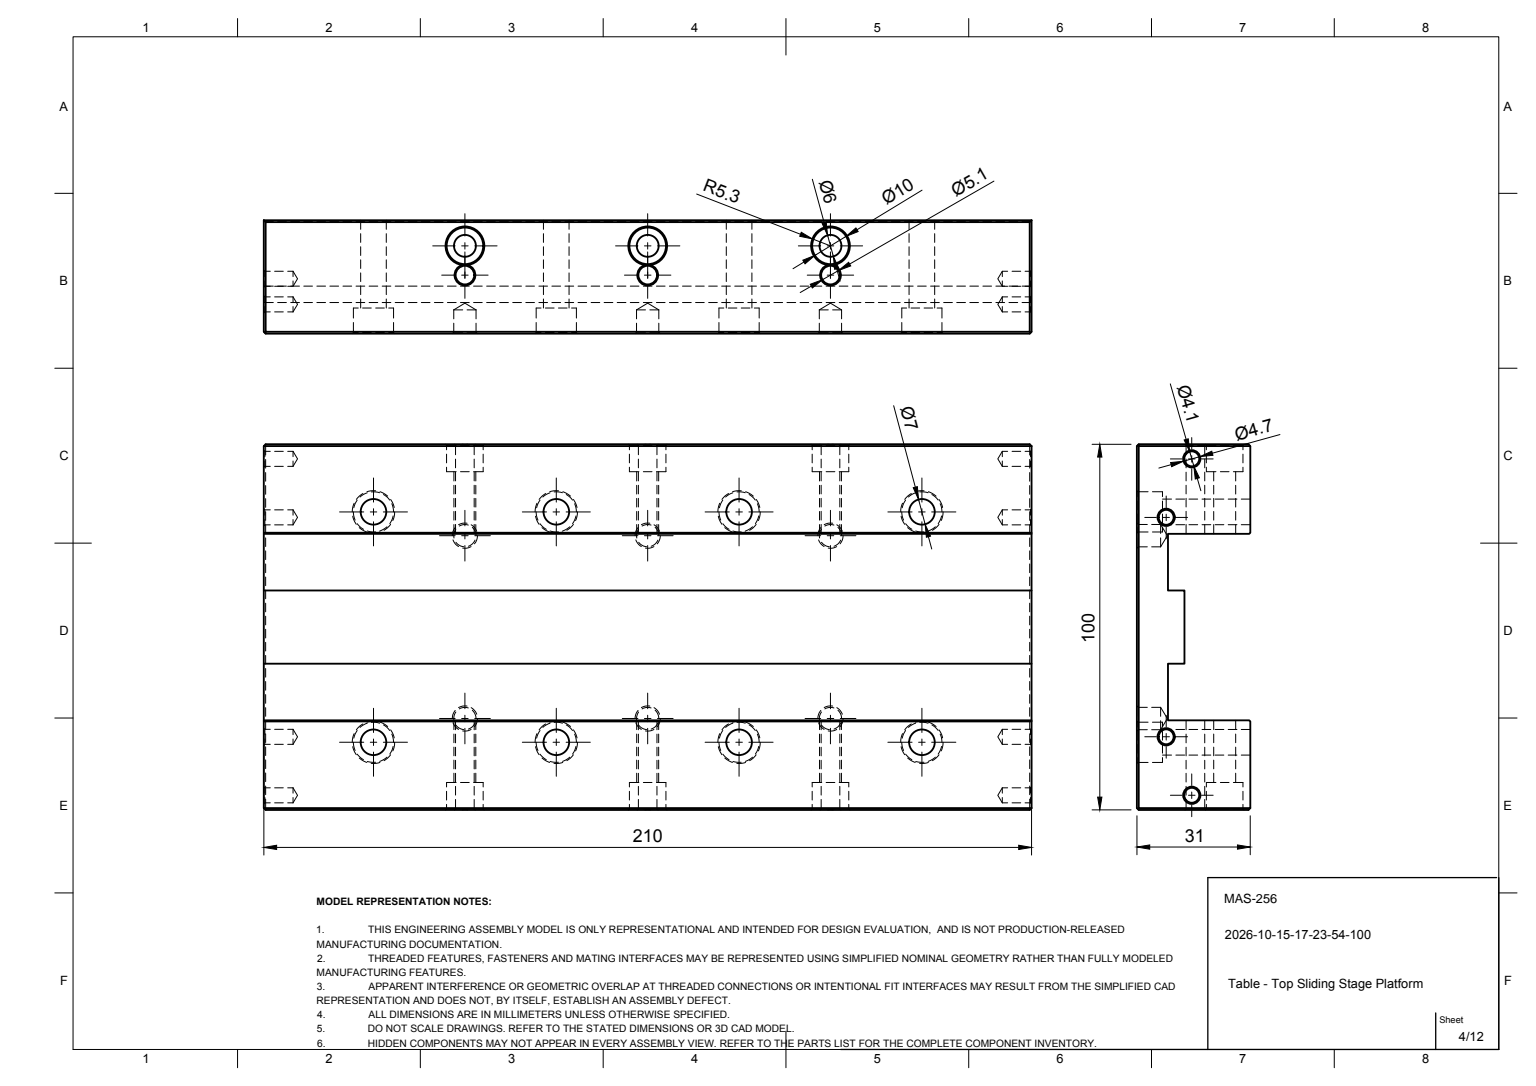
ISO-10303-21;
HEADER;
/* Generated by software containing ST-Developer
 * from STEP Tools, Inc. (www.steptools.com) 
 */

FILE_DESCRIPTION(
/* description */ (''),
/* implementation_level */ '2;1');

FILE_NAME(
/* name */ 'Table - Top Sliding Stage Platform.step',
/* time_stamp */ '2026-10-14T18:40:07-07:00',
/* author */ (''),
/* organization */ (''),
/* preprocessor_version */ 'ST-DEVELOPER v20.2',
/* originating_system */ 'Autodesk Translation Framework v15.15.0.0',
/* authorisation */ '');

FILE_SCHEMA (('AUTOMOTIVE_DESIGN { 1 0 10303 214 3 1 1 }'));
ENDSEC;

DATA;
#10=MECHANICAL_DESIGN_GEOMETRIC_PRESENTATION_REPRESENTATION('',(#832),#81040);
#402=B_SPLINE_CURVE_WITH_KNOTS('',3,(#20931,#20932,#20933,#20934,#20935,
#20936),.UNSPECIFIED.,.F.,.F.,(4,2,4),(1.66095691430957,1.73342009736541,
1.80588328042126),.UNSPECIFIED.);
#403=B_SPLINE_CURVE_WITH_KNOTS('',3,(#20957,#20958,#20959,#20960,#20961,
#20962),.UNSPECIFIED.,.F.,.F.,(4,2,4),(1.66095691430954,1.73342009736538,
1.80588328042123),.UNSPECIFIED.);
#404=B_SPLINE_CURVE_WITH_KNOTS('',3,(#20983,#20984,#20985,#20986,#20987,
#20988),.UNSPECIFIED.,.F.,.F.,(4,2,4),(1.66095691430954,1.73342009736541,
1.80588328042128),.UNSPECIFIED.);
#405=B_SPLINE_CURVE_WITH_KNOTS('',3,(#21051,#21052,#21053,#21054,#21055,
#21056),.UNSPECIFIED.,.F.,.F.,(4,2,4),(1.66095691430955,1.73342009736539,
1.80588328042123),.UNSPECIFIED.);
#406=B_SPLINE_CURVE_WITH_KNOTS('',3,(#21077,#21078,#21079,#21080,#21081,
#21082),.UNSPECIFIED.,.F.,.F.,(4,2,4),(1.66095691430953,1.73342009736537,
1.80588328042121),.UNSPECIFIED.);
#407=B_SPLINE_CURVE_WITH_KNOTS('',3,(#21103,#21104,#21105,#21106,#21107,
#21108),.UNSPECIFIED.,.F.,.F.,(4,2,4),(1.66095691430952,1.73342009736539,
1.80588328042126),.UNSPECIFIED.);
#812=SHAPE_REPRESENTATION_RELATIONSHIP('SRR','None',#81131,#822);
#822=ADVANCED_BREP_SHAPE_REPRESENTATION('',(#842),#81031);
#832=STYLED_ITEM('',(#81190),#842);
#842=MANIFOLD_SOLID_BREP('Body1',#15085);
#867=CYLINDRICAL_SURFACE('',#15336,2.55000000000001);
#868=CYLINDRICAL_SURFACE('',#15346,2.55000000000001);
#869=CYLINDRICAL_SURFACE('',#15356,2.55);
#870=CYLINDRICAL_SURFACE('',#15359,5.);
#871=CYLINDRICAL_SURFACE('',#15361,5.);
#872=CYLINDRICAL_SURFACE('',#15363,5.);
#873=CYLINDRICAL_SURFACE('',#15371,3.);
#874=CYLINDRICAL_SURFACE('',#15373,3.00000000000001);
#875=CYLINDRICAL_SURFACE('',#15375,3.00000000000001);
#876=CYLINDRICAL_SURFACE('',#15385,2.55000000000001);
#877=CYLINDRICAL_SURFACE('',#15395,2.55000000000001);
#878=CYLINDRICAL_SURFACE('',#15405,2.55);
#879=CYLINDRICAL_SURFACE('',#15408,5.);
#880=CYLINDRICAL_SURFACE('',#15410,5.);
#881=CYLINDRICAL_SURFACE('',#15412,5.);
#882=CYLINDRICAL_SURFACE('',#15420,3.);
#883=CYLINDRICAL_SURFACE('',#15422,3.00000000000001);
#884=CYLINDRICAL_SURFACE('',#15424,3.00000000000001);
#885=CYLINDRICAL_SURFACE('',#15433,2.05);
#886=CYLINDRICAL_SURFACE('',#15438,2.05);
#887=CYLINDRICAL_SURFACE('',#15443,2.05);
#888=CYLINDRICAL_SURFACE('',#15448,2.05);
#889=CYLINDRICAL_SURFACE('',#15462,2.05);
#890=CYLINDRICAL_SURFACE('',#15467,2.05);
#891=CYLINDRICAL_SURFACE('',#15472,2.05);
#892=CYLINDRICAL_SURFACE('',#15477,2.05);
#893=CYLINDRICAL_SURFACE('',#15501,3.05);
#894=CYLINDRICAL_SURFACE('',#15505,3.05);
#895=CYLINDRICAL_SURFACE('',#15509,3.05);
#896=CYLINDRICAL_SURFACE('',#15513,3.05);
#897=CYLINDRICAL_SURFACE('',#15517,3.05);
#898=CYLINDRICAL_SURFACE('',#15521,3.05);
#899=CYLINDRICAL_SURFACE('',#15531,5.50000000000001);
#900=CYLINDRICAL_SURFACE('',#15535,5.50000000000001);
#901=CYLINDRICAL_SURFACE('',#15539,5.5);
#902=CYLINDRICAL_SURFACE('',#15543,5.50000000000001);
#903=CYLINDRICAL_SURFACE('',#15547,5.5);
#904=CYLINDRICAL_SURFACE('',#15551,5.50000000000001);
#905=CYLINDRICAL_SURFACE('',#15555,5.50000000000001);
#906=CYLINDRICAL_SURFACE('',#15559,5.50000000000001);
#907=CYLINDRICAL_SURFACE('',#15577,3.50000000000001);
#908=CYLINDRICAL_SURFACE('',#15579,3.5);
#909=CYLINDRICAL_SURFACE('',#15581,3.5);
#910=CYLINDRICAL_SURFACE('',#15583,3.5);
#911=CYLINDRICAL_SURFACE('',#15585,3.5);
#912=CYLINDRICAL_SURFACE('',#15587,3.5);
#913=CYLINDRICAL_SURFACE('',#15589,3.5);
#914=CYLINDRICAL_SURFACE('',#15591,3.50000000000001);
#1107=FACE_BOUND('',#2455,.T.);
#1108=FACE_BOUND('',#2456,.T.);
#1109=FACE_BOUND('',#2457,.T.);
#1110=FACE_BOUND('',#2462,.T.);
#1111=FACE_BOUND('',#2464,.T.);
#1112=FACE_BOUND('',#2466,.T.);
#1113=FACE_BOUND('',#2480,.T.);
#1114=FACE_BOUND('',#2481,.T.);
#1115=FACE_BOUND('',#2482,.T.);
#1116=FACE_BOUND('',#2487,.T.);
#1117=FACE_BOUND('',#2489,.T.);
#1118=FACE_BOUND('',#2491,.T.);
#1119=FACE_BOUND('',#2497,.T.);
#1120=FACE_BOUND('',#2498,.T.);
#1121=FACE_BOUND('',#2499,.T.);
#1122=FACE_BOUND('',#2500,.T.);
#1123=FACE_BOUND('',#2514,.T.);
#1124=FACE_BOUND('',#2515,.T.);
#1125=FACE_BOUND('',#2516,.T.);
#1126=FACE_BOUND('',#2517,.T.);
#1127=FACE_BOUND('',#2531,.T.);
#1128=FACE_BOUND('',#2532,.T.);
#1129=FACE_BOUND('',#2533,.T.);
#1130=FACE_BOUND('',#2534,.T.);
#1131=FACE_BOUND('',#2535,.T.);
#1132=FACE_BOUND('',#2536,.T.);
#1133=FACE_BOUND('',#2537,.T.);
#1134=FACE_BOUND('',#2538,.T.);
#1135=FACE_BOUND('',#2539,.T.);
#1136=FACE_BOUND('',#2540,.T.);
#1137=FACE_BOUND('',#2541,.T.);
#1138=FACE_BOUND('',#2542,.T.);
#1139=FACE_BOUND('',#2543,.T.);
#1140=FACE_BOUND('',#2544,.T.);
#1141=FACE_BOUND('',#2579,.T.);
#1142=FACE_BOUND('',#2581,.T.);
#1143=FACE_BOUND('',#2583,.T.);
#1144=FACE_BOUND('',#2585,.T.);
#1145=FACE_BOUND('',#2587,.T.);
#1146=FACE_BOUND('',#2589,.T.);
#1147=FACE_BOUND('',#2591,.T.);
#1148=FACE_BOUND('',#2593,.T.);
#1149=FACE_BOUND('',#2613,.T.);
#1150=FACE_BOUND('',#2614,.T.);
#1151=FACE_BOUND('',#2615,.T.);
#1152=FACE_BOUND('',#2616,.T.);
#1153=FACE_BOUND('',#2619,.T.);
#1154=FACE_BOUND('',#2620,.T.);
#1155=FACE_BOUND('',#2621,.T.);
#1156=FACE_BOUND('',#2622,.T.);
#1157=FACE_BOUND('',#2623,.T.);
#1158=FACE_BOUND('',#2624,.T.);
#1159=FACE_BOUND('',#2627,.T.);
#1160=FACE_BOUND('',#2628,.T.);
#1161=FACE_BOUND('',#2629,.T.);
#1162=FACE_BOUND('',#2630,.T.);
#1163=FACE_BOUND('',#2632,.T.);
#1164=FACE_BOUND('',#2633,.T.);
#1165=FACE_BOUND('',#2634,.T.);
#1166=FACE_BOUND('',#2635,.T.);
#1167=FACE_BOUND('',#2636,.T.);
#1168=FACE_BOUND('',#2637,.T.);
#1243=PLANE('',#15358);
#1244=PLANE('',#15365);
#1245=PLANE('',#15367);
#1246=PLANE('',#15369);
#1247=PLANE('',#15407);
#1248=PLANE('',#15414);
#1249=PLANE('',#15416);
#1250=PLANE('',#15418);
#1251=PLANE('',#15429);
#1252=PLANE('',#15458);
#1253=PLANE('',#15487);
#1254=PLANE('',#15561);
#1255=PLANE('',#15563);
#1256=PLANE('',#15565);
#1257=PLANE('',#15567);
#1258=PLANE('',#15569);
#1259=PLANE('',#15571);
#1260=PLANE('',#15573);
#1261=PLANE('',#15575);
#1262=PLANE('',#15593);
#1263=PLANE('',#15594);
#1264=PLANE('',#15595);
#1265=PLANE('',#15596);
#1266=PLANE('',#15597);
#1267=PLANE('',#15598);
#1268=PLANE('',#15599);
#1269=PLANE('',#15600);
#1270=PLANE('',#15601);
#1271=PLANE('',#15602);
#1272=PLANE('',#15603);
#1273=PLANE('',#15604);
#1274=PLANE('',#15605);
#1275=PLANE('',#15606);
#1276=PLANE('',#15607);
#1277=PLANE('',#15608);
#1278=PLANE('',#15609);
#1279=PLANE('',#15610);
#1280=PLANE('',#15611);
#1281=PLANE('',#15612);
#1282=PLANE('',#15613);
#1678=FACE_OUTER_BOUND('',#2445,.T.);
#1679=FACE_OUTER_BOUND('',#2446,.T.);
#1680=FACE_OUTER_BOUND('',#2447,.T.);
#1681=FACE_OUTER_BOUND('',#2448,.T.);
#1682=FACE_OUTER_BOUND('',#2449,.T.);
#1683=FACE_OUTER_BOUND('',#2450,.T.);
#1684=FACE_OUTER_BOUND('',#2451,.T.);
#1685=FACE_OUTER_BOUND('',#2452,.T.);
#1686=FACE_OUTER_BOUND('',#2453,.T.);
#1687=FACE_OUTER_BOUND('',#2454,.T.);
#1688=FACE_OUTER_BOUND('',#2458,.T.);
#1689=FACE_OUTER_BOUND('',#2459,.T.);
#1690=FACE_OUTER_BOUND('',#2460,.T.);
#1691=FACE_OUTER_BOUND('',#2461,.T.);
#1692=FACE_OUTER_BOUND('',#2463,.T.);
#1693=FACE_OUTER_BOUND('',#2465,.T.);
#1694=FACE_OUTER_BOUND('',#2467,.T.);
#1695=FACE_OUTER_BOUND('',#2468,.T.);
#1696=FACE_OUTER_BOUND('',#2469,.T.);
#1697=FACE_OUTER_BOUND('',#2470,.T.);
#1698=FACE_OUTER_BOUND('',#2471,.T.);
#1699=FACE_OUTER_BOUND('',#2472,.T.);
#1700=FACE_OUTER_BOUND('',#2473,.T.);
#1701=FACE_OUTER_BOUND('',#2474,.T.);
#1702=FACE_OUTER_BOUND('',#2475,.T.);
#1703=FACE_OUTER_BOUND('',#2476,.T.);
#1704=FACE_OUTER_BOUND('',#2477,.T.);
#1705=FACE_OUTER_BOUND('',#2478,.T.);
#1706=FACE_OUTER_BOUND('',#2479,.T.);
#1707=FACE_OUTER_BOUND('',#2483,.T.);
#1708=FACE_OUTER_BOUND('',#2484,.T.);
#1709=FACE_OUTER_BOUND('',#2485,.T.);
#1710=FACE_OUTER_BOUND('',#2486,.T.);
#1711=FACE_OUTER_BOUND('',#2488,.T.);
#1712=FACE_OUTER_BOUND('',#2490,.T.);
#1713=FACE_OUTER_BOUND('',#2492,.T.);
#1714=FACE_OUTER_BOUND('',#2493,.T.);
#1715=FACE_OUTER_BOUND('',#2494,.T.);
#1716=FACE_OUTER_BOUND('',#2495,.T.);
#1717=FACE_OUTER_BOUND('',#2496,.T.);
#1718=FACE_OUTER_BOUND('',#2501,.T.);
#1719=FACE_OUTER_BOUND('',#2502,.T.);
#1720=FACE_OUTER_BOUND('',#2503,.T.);
#1721=FACE_OUTER_BOUND('',#2504,.T.);
#1722=FACE_OUTER_BOUND('',#2505,.T.);
#1723=FACE_OUTER_BOUND('',#2506,.T.);
#1724=FACE_OUTER_BOUND('',#2507,.T.);
#1725=FACE_OUTER_BOUND('',#2508,.T.);
#1726=FACE_OUTER_BOUND('',#2509,.T.);
#1727=FACE_OUTER_BOUND('',#2510,.T.);
#1728=FACE_OUTER_BOUND('',#2511,.T.);
#1729=FACE_OUTER_BOUND('',#2512,.T.);
#1730=FACE_OUTER_BOUND('',#2513,.T.);
#1731=FACE_OUTER_BOUND('',#2518,.T.);
#1732=FACE_OUTER_BOUND('',#2519,.T.);
#1733=FACE_OUTER_BOUND('',#2520,.T.);
#1734=FACE_OUTER_BOUND('',#2521,.T.);
#1735=FACE_OUTER_BOUND('',#2522,.T.);
#1736=FACE_OUTER_BOUND('',#2523,.T.);
#1737=FACE_OUTER_BOUND('',#2524,.T.);
#1738=FACE_OUTER_BOUND('',#2525,.T.);
#1739=FACE_OUTER_BOUND('',#2526,.T.);
#1740=FACE_OUTER_BOUND('',#2527,.T.);
#1741=FACE_OUTER_BOUND('',#2528,.T.);
#1742=FACE_OUTER_BOUND('',#2529,.T.);
#1743=FACE_OUTER_BOUND('',#2530,.T.);
#1744=FACE_OUTER_BOUND('',#2545,.T.);
#1745=FACE_OUTER_BOUND('',#2546,.T.);
#1746=FACE_OUTER_BOUND('',#2547,.T.);
#1747=FACE_OUTER_BOUND('',#2548,.T.);
#1748=FACE_OUTER_BOUND('',#2549,.T.);
#1749=FACE_OUTER_BOUND('',#2550,.T.);
#1750=FACE_OUTER_BOUND('',#2551,.T.);
#1751=FACE_OUTER_BOUND('',#2552,.T.);
#1752=FACE_OUTER_BOUND('',#2553,.T.);
#1753=FACE_OUTER_BOUND('',#2554,.T.);
#1754=FACE_OUTER_BOUND('',#2555,.T.);
#1755=FACE_OUTER_BOUND('',#2556,.T.);
#1756=FACE_OUTER_BOUND('',#2557,.T.);
#1757=FACE_OUTER_BOUND('',#2558,.T.);
#1758=FACE_OUTER_BOUND('',#2559,.T.);
#1759=FACE_OUTER_BOUND('',#2560,.T.);
#1760=FACE_OUTER_BOUND('',#2561,.T.);
#1761=FACE_OUTER_BOUND('',#2562,.T.);
#1762=FACE_OUTER_BOUND('',#2563,.T.);
#1763=FACE_OUTER_BOUND('',#2564,.T.);
#1764=FACE_OUTER_BOUND('',#2565,.T.);
#1765=FACE_OUTER_BOUND('',#2566,.T.);
#1766=FACE_OUTER_BOUND('',#2567,.T.);
#1767=FACE_OUTER_BOUND('',#2568,.T.);
#1768=FACE_OUTER_BOUND('',#2569,.T.);
#1769=FACE_OUTER_BOUND('',#2570,.T.);
#1770=FACE_OUTER_BOUND('',#2571,.T.);
#1771=FACE_OUTER_BOUND('',#2572,.T.);
#1772=FACE_OUTER_BOUND('',#2573,.T.);
#1773=FACE_OUTER_BOUND('',#2574,.T.);
#1774=FACE_OUTER_BOUND('',#2575,.T.);
#1775=FACE_OUTER_BOUND('',#2576,.T.);
#1776=FACE_OUTER_BOUND('',#2577,.T.);
#1777=FACE_OUTER_BOUND('',#2578,.T.);
#1778=FACE_OUTER_BOUND('',#2580,.T.);
#1779=FACE_OUTER_BOUND('',#2582,.T.);
#1780=FACE_OUTER_BOUND('',#2584,.T.);
#1781=FACE_OUTER_BOUND('',#2586,.T.);
#1782=FACE_OUTER_BOUND('',#2588,.T.);
#1783=FACE_OUTER_BOUND('',#2590,.T.);
#1784=FACE_OUTER_BOUND('',#2592,.T.);
#1785=FACE_OUTER_BOUND('',#2594,.T.);
#1786=FACE_OUTER_BOUND('',#2595,.T.);
#1787=FACE_OUTER_BOUND('',#2596,.T.);
#1788=FACE_OUTER_BOUND('',#2597,.T.);
#1789=FACE_OUTER_BOUND('',#2598,.T.);
#1790=FACE_OUTER_BOUND('',#2599,.T.);
#1791=FACE_OUTER_BOUND('',#2600,.T.);
#1792=FACE_OUTER_BOUND('',#2601,.T.);
#1793=FACE_OUTER_BOUND('',#2602,.T.);
#1794=FACE_OUTER_BOUND('',#2603,.T.);
#1795=FACE_OUTER_BOUND('',#2604,.T.);
#1796=FACE_OUTER_BOUND('',#2605,.T.);
#1797=FACE_OUTER_BOUND('',#2606,.T.);
#1798=FACE_OUTER_BOUND('',#2607,.T.);
#1799=FACE_OUTER_BOUND('',#2608,.T.);
#1800=FACE_OUTER_BOUND('',#2609,.T.);
#1801=FACE_OUTER_BOUND('',#2610,.T.);
#1802=FACE_OUTER_BOUND('',#2611,.T.);
#1803=FACE_OUTER_BOUND('',#2612,.T.);
#1804=FACE_OUTER_BOUND('',#2617,.T.);
#1805=FACE_OUTER_BOUND('',#2618,.T.);
#1806=FACE_OUTER_BOUND('',#2625,.T.);
#1807=FACE_OUTER_BOUND('',#2626,.T.);
#1808=FACE_OUTER_BOUND('',#2631,.T.);
#1809=FACE_OUTER_BOUND('',#2638,.T.);
#1810=FACE_OUTER_BOUND('',#2639,.T.);
#1811=FACE_OUTER_BOUND('',#2640,.T.);
#1812=FACE_OUTER_BOUND('',#2641,.T.);
#1813=FACE_OUTER_BOUND('',#2642,.T.);
#2445=EDGE_LOOP('',(#10130,#10131,#10132,#10133,#10134,#10135));
#2446=EDGE_LOOP('',(#10136,#10137,#10138,#10139,#10140,#10141));
#2447=EDGE_LOOP('',(#10142,#10143,#10144,#10145));
#2448=EDGE_LOOP('',(#10146,#10147,#10148,#10149,#10150,#10151));
#2449=EDGE_LOOP('',(#10152,#10153,#10154,#10155,#10156,#10157));
#2450=EDGE_LOOP('',(#10158,#10159,#10160,#10161));
#2451=EDGE_LOOP('',(#10162,#10163,#10164,#10165,#10166,#10167));
#2452=EDGE_LOOP('',(#10168,#10169,#10170,#10171,#10172,#10173));
#2453=EDGE_LOOP('',(#10174,#10175,#10176,#10177));
#2454=EDGE_LOOP('',(#10178,#10179,#10180,#10181));
#2455=EDGE_LOOP('',(#10182,#10183,#10184,#10185));
#2456=EDGE_LOOP('',(#10186,#10187,#10188,#10189));
#2457=EDGE_LOOP('',(#10190,#10191,#10192,#10193));
#2458=EDGE_LOOP('',(#10194,#10195,#10196,#10197));
#2459=EDGE_LOOP('',(#10198,#10199,#10200,#10201));
#2460=EDGE_LOOP('',(#10202,#10203,#10204,#10205));
#2461=EDGE_LOOP('',(#10206));
#2462=EDGE_LOOP('',(#10207));
#2463=EDGE_LOOP('',(#10208));
#2464=EDGE_LOOP('',(#10209));
#2465=EDGE_LOOP('',(#10210));
#2466=EDGE_LOOP('',(#10211));
#2467=EDGE_LOOP('',(#10212,#10213,#10214,#10215));
#2468=EDGE_LOOP('',(#10216,#10217,#10218,#10219));
#2469=EDGE_LOOP('',(#10220,#10221,#10222,#10223));
#2470=EDGE_LOOP('',(#10224,#10225,#10226,#10227,#10228,#10229));
#2471=EDGE_LOOP('',(#10230,#10231,#10232,#10233,#10234,#10235));
#2472=EDGE_LOOP('',(#10236,#10237,#10238,#10239));
#2473=EDGE_LOOP('',(#10240,#10241,#10242,#10243,#10244,#10245));
#2474=EDGE_LOOP('',(#10246,#10247,#10248,#10249,#10250,#10251));
#2475=EDGE_LOOP('',(#10252,#10253,#10254,#10255));
#2476=EDGE_LOOP('',(#10256,#10257,#10258,#10259,#10260,#10261));
#2477=EDGE_LOOP('',(#10262,#10263,#10264,#10265,#10266,#10267));
#2478=EDGE_LOOP('',(#10268,#10269,#10270,#10271));
#2479=EDGE_LOOP('',(#10272,#10273,#10274,#10275));
#2480=EDGE_LOOP('',(#10276,#10277,#10278,#10279));
#2481=EDGE_LOOP('',(#10280,#10281,#10282,#10283));
#2482=EDGE_LOOP('',(#10284,#10285,#10286,#10287));
#2483=EDGE_LOOP('',(#10288,#10289,#10290,#10291));
#2484=EDGE_LOOP('',(#10292,#10293,#10294,#10295));
#2485=EDGE_LOOP('',(#10296,#10297,#10298,#10299));
#2486=EDGE_LOOP('',(#10300));
#2487=EDGE_LOOP('',(#10301));
#2488=EDGE_LOOP('',(#10302));
#2489=EDGE_LOOP('',(#10303));
#2490=EDGE_LOOP('',(#10304));
#2491=EDGE_LOOP('',(#10305));
#2492=EDGE_LOOP('',(#10306,#10307,#10308,#10309));
#2493=EDGE_LOOP('',(#10310,#10311,#10312,#10313));
#2494=EDGE_LOOP('',(#10314,#10315,#10316,#10317));
#2495=EDGE_LOOP('',(#10318,#10319,#10320,#10321));
#2496=EDGE_LOOP('',(#10322,#10323,#10324,#10325,#10326,#10327,#10328,#10329,
#10330,#10331,#10332,#10333,#10334,#10335));
#2497=EDGE_LOOP('',(#10336));
#2498=EDGE_LOOP('',(#10337));
#2499=EDGE_LOOP('',(#10338));
#2500=EDGE_LOOP('',(#10339));
#2501=EDGE_LOOP('',(#10340,#10341,#10342,#10343,#10344));
#2502=EDGE_LOOP('',(#10345,#10346,#10347,#10348));
#2503=EDGE_LOOP('',(#10349,#10350,#10351,#10352,#10353));
#2504=EDGE_LOOP('',(#10354,#10355,#10356,#10357));
#2505=EDGE_LOOP('',(#10358,#10359,#10360,#10361,#10362));
#2506=EDGE_LOOP('',(#10363,#10364,#10365,#10366));
#2507=EDGE_LOOP('',(#10367,#10368,#10369,#10370,#10371));
#2508=EDGE_LOOP('',(#10372,#10373,#10374,#10375));
#2509=EDGE_LOOP('',(#10376,#10377,#10378,#10379));
#2510=EDGE_LOOP('',(#10380,#10381,#10382,#10383));
#2511=EDGE_LOOP('',(#10384,#10385,#10386,#10387));
#2512=EDGE_LOOP('',(#10388,#10389,#10390,#10391));
#2513=EDGE_LOOP('',(#10392,#10393,#10394,#10395,#10396,#10397,#10398,#10399,
#10400,#10401,#10402,#10403,#10404,#10405));
#2514=EDGE_LOOP('',(#10406));
#2515=EDGE_LOOP('',(#10407));
#2516=EDGE_LOOP('',(#10408));
#2517=EDGE_LOOP('',(#10409));
#2518=EDGE_LOOP('',(#10410,#10411,#10412,#10413,#10414));
#2519=EDGE_LOOP('',(#10415,#10416,#10417,#10418));
#2520=EDGE_LOOP('',(#10419,#10420,#10421,#10422,#10423));
#2521=EDGE_LOOP('',(#10424,#10425,#10426,#10427));
#2522=EDGE_LOOP('',(#10428,#10429,#10430,#10431,#10432));
#2523=EDGE_LOOP('',(#10433,#10434,#10435,#10436));
#2524=EDGE_LOOP('',(#10437,#10438,#10439,#10440,#10441));
#2525=EDGE_LOOP('',(#10442,#10443,#10444,#10445));
#2526=EDGE_LOOP('',(#10446,#10447,#10448,#10449));
#2527=EDGE_LOOP('',(#10450,#10451,#10452,#10453));
#2528=EDGE_LOOP('',(#10454,#10455,#10456,#10457));
#2529=EDGE_LOOP('',(#10458,#10459,#10460,#10461));
#2530=EDGE_LOOP('',(#10462,#10463,#10464,#10465));
#2531=EDGE_LOOP('',(#10466));
#2532=EDGE_LOOP('',(#10467));
#2533=EDGE_LOOP('',(#10468));
#2534=EDGE_LOOP('',(#10469));
#2535=EDGE_LOOP('',(#10470));
#2536=EDGE_LOOP('',(#10471));
#2537=EDGE_LOOP('',(#10472));
#2538=EDGE_LOOP('',(#10473));
#2539=EDGE_LOOP('',(#10474));
#2540=EDGE_LOOP('',(#10475));
#2541=EDGE_LOOP('',(#10476));
#2542=EDGE_LOOP('',(#10477));
#2543=EDGE_LOOP('',(#10478));
#2544=EDGE_LOOP('',(#10479));
#2545=EDGE_LOOP('',(#10480,#10481,#10482,#10483));
#2546=EDGE_LOOP('',(#10484,#10485,#10486,#10487));
#2547=EDGE_LOOP('',(#10488,#10489,#10490,#10491));
#2548=EDGE_LOOP('',(#10492,#10493,#10494,#10495));
#2549=EDGE_LOOP('',(#10496,#10497,#10498,#10499));
#2550=EDGE_LOOP('',(#10500,#10501,#10502,#10503));
#2551=EDGE_LOOP('',(#10504,#10505,#10506,#10507));
#2552=EDGE_LOOP('',(#10508,#10509,#10510,#10511));
#2553=EDGE_LOOP('',(#10512,#10513,#10514,#10515));
#2554=EDGE_LOOP('',(#10516,#10517,#10518,#10519));
#2555=EDGE_LOOP('',(#10520,#10521,#10522,#10523));
#2556=EDGE_LOOP('',(#10524,#10525,#10526));
#2557=EDGE_LOOP('',(#10527,#10528,#10529));
#2558=EDGE_LOOP('',(#10530,#10531,#10532));
#2559=EDGE_LOOP('',(#10533,#10534,#10535));
#2560=EDGE_LOOP('',(#10536,#10537,#10538));
#2561=EDGE_LOOP('',(#10539,#10540,#10541));
#2562=EDGE_LOOP('',(#10542,#10543,#10544,#10545));
#2563=EDGE_LOOP('',(#10546,#10547,#10548,#10549));
#2564=EDGE_LOOP('',(#10550,#10551,#10552,#10553));
#2565=EDGE_LOOP('',(#10554,#10555,#10556,#10557));
#2566=EDGE_LOOP('',(#10558,#10559,#10560,#10561));
#2567=EDGE_LOOP('',(#10562,#10563,#10564,#10565));
#2568=EDGE_LOOP('',(#10566,#10567,#10568,#10569));
#2569=EDGE_LOOP('',(#10570,#10571,#10572,#10573));
#2570=EDGE_LOOP('',(#10574,#10575,#10576,#10577));
#2571=EDGE_LOOP('',(#10578,#10579,#10580,#10581));
#2572=EDGE_LOOP('',(#10582,#10583,#10584,#10585));
#2573=EDGE_LOOP('',(#10586,#10587,#10588,#10589));
#2574=EDGE_LOOP('',(#10590,#10591,#10592,#10593));
#2575=EDGE_LOOP('',(#10594,#10595,#10596,#10597));
#2576=EDGE_LOOP('',(#10598,#10599,#10600,#10601));
#2577=EDGE_LOOP('',(#10602,#10603,#10604,#10605));
#2578=EDGE_LOOP('',(#10606));
#2579=EDGE_LOOP('',(#10607));
#2580=EDGE_LOOP('',(#10608));
#2581=EDGE_LOOP('',(#10609));
#2582=EDGE_LOOP('',(#10610));
#2583=EDGE_LOOP('',(#10611));
#2584=EDGE_LOOP('',(#10612));
#2585=EDGE_LOOP('',(#10613));
#2586=EDGE_LOOP('',(#10614));
#2587=EDGE_LOOP('',(#10615));
#2588=EDGE_LOOP('',(#10616));
#2589=EDGE_LOOP('',(#10617));
#2590=EDGE_LOOP('',(#10618));
#2591=EDGE_LOOP('',(#10619));
#2592=EDGE_LOOP('',(#10620));
#2593=EDGE_LOOP('',(#10621));
#2594=EDGE_LOOP('',(#10622,#10623,#10624,#10625));
#2595=EDGE_LOOP('',(#10626,#10627,#10628,#10629));
#2596=EDGE_LOOP('',(#10630,#10631,#10632,#10633));
#2597=EDGE_LOOP('',(#10634,#10635,#10636,#10637));
#2598=EDGE_LOOP('',(#10638,#10639,#10640,#10641));
#2599=EDGE_LOOP('',(#10642,#10643,#10644,#10645));
#2600=EDGE_LOOP('',(#10646,#10647,#10648,#10649));
#2601=EDGE_LOOP('',(#10650,#10651,#10652,#10653));
#2602=EDGE_LOOP('',(#10654,#10655,#10656,#10657,#10658));
#2603=EDGE_LOOP('',(#10659,#10660,#10661,#10662,#10663,#10664));
#2604=EDGE_LOOP('',(#10665,#10666,#10667,#10668));
#2605=EDGE_LOOP('',(#10669,#10670,#10671,#10672,#10673,#10674));
#2606=EDGE_LOOP('',(#10675,#10676,#10677,#10678,#10679));
#2607=EDGE_LOOP('',(#10680,#10681,#10682,#10683,#10684));
#2608=EDGE_LOOP('',(#10685,#10686,#10687,#10688,#10689,#10690));
#2609=EDGE_LOOP('',(#10691,#10692,#10693,#10694,#10695,#10696));
#2610=EDGE_LOOP('',(#10697,#10698,#10699,#10700,#10701));
#2611=EDGE_LOOP('',(#10702,#10703,#10704,#10705));
#2612=EDGE_LOOP('',(#10706,#10707,#10708,#10709));
#2613=EDGE_LOOP('',(#10710));
#2614=EDGE_LOOP('',(#10711));
#2615=EDGE_LOOP('',(#10712));
#2616=EDGE_LOOP('',(#10713));
#2617=EDGE_LOOP('',(#10714,#10715,#10716,#10717));
#2618=EDGE_LOOP('',(#10718,#10719,#10720,#10721));
#2619=EDGE_LOOP('',(#10722));
#2620=EDGE_LOOP('',(#10723));
#2621=EDGE_LOOP('',(#10724));
#2622=EDGE_LOOP('',(#10725));
#2623=EDGE_LOOP('',(#10726));
#2624=EDGE_LOOP('',(#10727));
#2625=EDGE_LOOP('',(#10728,#10729,#10730,#10731));
#2626=EDGE_LOOP('',(#10732,#10733,#10734,#10735));
#2627=EDGE_LOOP('',(#10736));
#2628=EDGE_LOOP('',(#10737));
#2629=EDGE_LOOP('',(#10738));
#2630=EDGE_LOOP('',(#10739));
#2631=EDGE_LOOP('',(#10740,#10741,#10742,#10743));
#2632=EDGE_LOOP('',(#10744));
#2633=EDGE_LOOP('',(#10745));
#2634=EDGE_LOOP('',(#10746));
#2635=EDGE_LOOP('',(#10747));
#2636=EDGE_LOOP('',(#10748));
#2637=EDGE_LOOP('',(#10749));
#2638=EDGE_LOOP('',(#10750,#10751,#10752,#10753));
#2639=EDGE_LOOP('',(#10754,#10755,#10756,#10757));
#2640=EDGE_LOOP('',(#10758,#10759,#10760,#10761));
#2641=EDGE_LOOP('',(#10762,#10763,#10764,#10765));
#2642=EDGE_LOOP('',(#10766,#10767,#10768,#10769));
#3346=LINE('',#20927,#4458);
#3347=LINE('',#20942,#4459);
#3348=LINE('',#20947,#4460);
#3349=LINE('',#20953,#4461);
#3350=LINE('',#20968,#4462);
#3351=LINE('',#20973,#4463);
#3352=LINE('',#20979,#4464);
#3353=LINE('',#20994,#4465);
#3354=LINE('',#20999,#4466);
#3355=LINE('',#21004,#4467);
#3356=LINE('',#21006,#4468);
#3357=LINE('',#21008,#4469);
#3358=LINE('',#21009,#4470);
#3359=LINE('',#21012,#4471);
#3360=LINE('',#21016,#4472);
#3361=LINE('',#21020,#4473);
#3362=LINE('',#21033,#4474);
#3363=LINE('',#21037,#4475);
#3364=LINE('',#21041,#4476);
#3365=LINE('',#21047,#4477);
#3366=LINE('',#21062,#4478);
#3367=LINE('',#21067,#4479);
#3368=LINE('',#21073,#4480);
#3369=LINE('',#21088,#4481);
#3370=LINE('',#21093,#4482);
#3371=LINE('',#21099,#4483);
#3372=LINE('',#21114,#4484);
#3373=LINE('',#21119,#4485);
#3374=LINE('',#21124,#4486);
#3375=LINE('',#21126,#4487);
#3376=LINE('',#21128,#4488);
#3377=LINE('',#21129,#4489);
#3378=LINE('',#21132,#4490);
#3379=LINE('',#21136,#4491);
#3380=LINE('',#21140,#4492);
#3381=LINE('',#21153,#4493);
#3382=LINE('',#21157,#4494);
#3383=LINE('',#21161,#4495);
#3384=LINE('',#21167,#4496);
#3385=LINE('',#21172,#4497);
#3386=LINE('',#21174,#4498);
#3387=LINE('',#21176,#4499);
#3388=LINE('',#21178,#4500);
#3389=LINE('',#21180,#4501);
#3390=LINE('',#21182,#4502);
#3391=LINE('',#21184,#4503);
#3392=LINE('',#21186,#4504);
#3393=LINE('',#21188,#4505);
#3394=LINE('',#21190,#4506);
#3395=LINE('',#21192,#4507);
#3396=LINE('',#21194,#4508);
#3397=LINE('',#21196,#4509);
#3398=LINE('',#21197,#4510);
#3399=LINE('',#21206,#4511);
#3400=LINE('',#21213,#4512);
#3401=LINE('',#21216,#4513);
#3402=LINE('',#21223,#4514);
#3403=LINE('',#21226,#4515);
#3404=LINE('',#21233,#4516);
#3405=LINE('',#21236,#4517);
#3406=LINE('',#21242,#4518);
#3407=LINE('',#21245,#4519);
#3408=LINE('',#21248,#4520);
#3409=LINE('',#21251,#4521);
#3410=LINE('',#21256,#4522);
#3411=LINE('',#21261,#4523);
#3412=LINE('',#21263,#4524);
#3413=LINE('',#21265,#4525);
#3414=LINE('',#21267,#4526);
#3415=LINE('',#21269,#4527);
#3416=LINE('',#21271,#4528);
#3417=LINE('',#21273,#4529);
#3418=LINE('',#21275,#4530);
#3419=LINE('',#21277,#4531);
#3420=LINE('',#21279,#4532);
#3421=LINE('',#21281,#4533);
#3422=LINE('',#21283,#4534);
#3423=LINE('',#21285,#4535);
#3424=LINE('',#21286,#4536);
#3425=LINE('',#21295,#4537);
#3426=LINE('',#21302,#4538);
#3427=LINE('',#21305,#4539);
#3428=LINE('',#21312,#4540);
#3429=LINE('',#21315,#4541);
#3430=LINE('',#21322,#4542);
#3431=LINE('',#21325,#4543);
#3432=LINE('',#21331,#4544);
#3433=LINE('',#21334,#4545);
#3434=LINE('',#21337,#4546);
#3435=LINE('',#21340,#4547);
#3436=LINE('',#21345,#4548);
#3437=LINE('',#21350,#4549);
#3438=LINE('',#21352,#4550);
#3439=LINE('',#21354,#4551);
#3440=LINE('',#21355,#4552);
#3441=LINE('',#21384,#4553);
#3442=LINE('',#21389,#4554);
#3443=LINE('',#21392,#4555);
#3444=LINE('',#21397,#4556);
#3445=LINE('',#21400,#4557);
#3446=LINE('',#21405,#4558);
#3447=LINE('',#21408,#4559);
#3448=LINE('',#21413,#4560);
#3449=LINE('',#21416,#4561);
#3450=LINE('',#21421,#4562);
#3451=LINE('',#21424,#4563);
#3452=LINE('',#21428,#4564);
#3453=LINE('',#21431,#4565);
#3454=LINE('',#21434,#4566);
#3455=LINE('',#21437,#4567);
#3456=LINE('',#21440,#4568);
#3457=LINE('',#21443,#4569);
#3458=LINE('',#21447,#4570);
#3459=LINE('',#21450,#4571);
#3460=LINE('',#21455,#4572);
#3461=LINE('',#21458,#4573);
#3462=LINE('',#21463,#4574);
#3463=LINE('',#21466,#4575);
#3464=LINE('',#21471,#4576);
#3465=LINE('',#21474,#4577);
#3466=LINE('',#21479,#4578);
#3467=LINE('',#21482,#4579);
#3468=LINE('',#21487,#4580);
#3469=LINE('',#21490,#4581);
#3470=LINE('',#21495,#4582);
#3471=LINE('',#21498,#4583);
#3472=LINE('',#21503,#4584);
#3473=LINE('',#21506,#4585);
#3474=LINE('',#21534,#4586);
#3475=LINE('',#21538,#4587);
#3476=LINE('',#21542,#4588);
#3477=LINE('',#21546,#4589);
#3478=LINE('',#21550,#4590);
#3479=LINE('',#21554,#4591);
#3480=LINE('',#21558,#4592);
#3481=LINE('',#21562,#4593);
#3482=LINE('',#21565,#4594);
#3483=LINE('',#21567,#4595);
#3484=LINE('',#21568,#4596);
#3485=LINE('',#21571,#4597);
#3486=LINE('',#21572,#4598);
#3487=LINE('',#21573,#4599);
#3488=LINE('',#21575,#4600);
#3489=LINE('',#21576,#4601);
#3490=LINE('',#21578,#4602);
#3491=LINE('',#21580,#4603);
#3492=LINE('',#21581,#4604);
#3493=LINE('',#21583,#4605);
#3494=LINE('',#21585,#4606);
#3495=LINE('',#21586,#4607);
#3496=LINE('',#21589,#4608);
#3497=LINE('',#21590,#4609);
#3498=LINE('',#21592,#4610);
#3499=LINE('',#21595,#4611);
#3500=LINE('',#21596,#4612);
#3501=LINE('',#21598,#4613);
#3502=LINE('',#21600,#4614);
#3503=LINE('',#21601,#4615);
#3504=LINE('',#21603,#4616);
#3505=LINE('',#21607,#4617);
#3506=LINE('',#21609,#4618);
#3507=LINE('',#21611,#4619);
#3508=LINE('',#21613,#4620);
#3509=LINE('',#21615,#4621);
#4458=VECTOR('',#16996,2.7);
#4459=VECTOR('',#17005,5.15000000000001);
#4460=VECTOR('',#17012,2.55000000000001);
#4461=VECTOR('',#17019,2.7);
#4462=VECTOR('',#17028,5.15);
#4463=VECTOR('',#17035,2.55000000000001);
#4464=VECTOR('',#17042,2.7);
#4465=VECTOR('',#17051,5.15);
#4466=VECTOR('',#17058,2.55);
#4467=VECTOR('',#17063,10.);
#4468=VECTOR('',#17064,10.);
#4469=VECTOR('',#17065,10.);
#4470=VECTOR('',#17066,10.);
#4471=VECTOR('',#17069,5.);
#4472=VECTOR('',#17074,5.);
#4473=VECTOR('',#17079,5.);
#4474=VECTOR('',#17096,3.);
#4475=VECTOR('',#17101,3.00000000000001);
#4476=VECTOR('',#17106,3.00000000000001);
#4477=VECTOR('',#17113,2.7);
#4478=VECTOR('',#17122,5.15000000000001);
#4479=VECTOR('',#17129,2.55000000000001);
#4480=VECTOR('',#17136,2.7);
#4481=VECTOR('',#17145,5.15);
#4482=VECTOR('',#17152,2.55000000000001);
#4483=VECTOR('',#17159,2.7);
#4484=VECTOR('',#17168,5.15);
#4485=VECTOR('',#17175,2.55);
#4486=VECTOR('',#17180,10.);
#4487=VECTOR('',#17181,10.);
#4488=VECTOR('',#17182,10.);
#4489=VECTOR('',#17183,10.);
#4490=VECTOR('',#17186,5.);
#4491=VECTOR('',#17191,5.);
#4492=VECTOR('',#17196,5.);
#4493=VECTOR('',#17213,3.);
#4494=VECTOR('',#17218,3.00000000000001);
#4495=VECTOR('',#17223,3.00000000000001);
#4496=VECTOR('',#17230,2.2);
#4497=VECTOR('',#17235,10.);
#4498=VECTOR('',#17236,10.);
#4499=VECTOR('',#17237,10.);
#4500=VECTOR('',#17238,10.);
#4501=VECTOR('',#17239,10.);
#4502=VECTOR('',#17240,10.);
#4503=VECTOR('',#17241,10.);
#4504=VECTOR('',#17242,10.);
#4505=VECTOR('',#17243,10.);
#4506=VECTOR('',#17244,10.);
#4507=VECTOR('',#17245,10.);
#4508=VECTOR('',#17246,10.);
#4509=VECTOR('',#17247,10.);
#4510=VECTOR('',#17248,10.);
#4511=VECTOR('',#17257,2.05);
#4512=VECTOR('',#17266,2.2);
#4513=VECTOR('',#17269,2.05);
#4514=VECTOR('',#17278,2.2);
#4515=VECTOR('',#17281,2.05);
#4516=VECTOR('',#17290,2.2);
#4517=VECTOR('',#17293,2.05);
#4518=VECTOR('',#17300,1.025);
#4519=VECTOR('',#17303,1.025);
#4520=VECTOR('',#17306,1.025);
#4521=VECTOR('',#17309,1.025);
#4522=VECTOR('',#17314,2.2);
#4523=VECTOR('',#17319,10.);
#4524=VECTOR('',#17320,10.);
#4525=VECTOR('',#17321,10.);
#4526=VECTOR('',#17322,10.);
#4527=VECTOR('',#17323,10.);
#4528=VECTOR('',#17324,10.);
#4529=VECTOR('',#17325,10.);
#4530=VECTOR('',#17326,10.);
#4531=VECTOR('',#17327,10.);
#4532=VECTOR('',#17328,10.);
#4533=VECTOR('',#17329,10.);
#4534=VECTOR('',#17330,10.);
#4535=VECTOR('',#17331,10.);
#4536=VECTOR('',#17332,10.);
#4537=VECTOR('',#17341,2.05);
#4538=VECTOR('',#17350,2.2);
#4539=VECTOR('',#17353,2.05);
#4540=VECTOR('',#17362,2.2);
#4541=VECTOR('',#17365,2.05);
#4542=VECTOR('',#17374,2.2);
#4543=VECTOR('',#17377,2.05);
#4544=VECTOR('',#17384,2.05);
#4545=VECTOR('',#17387,2.05);
#4546=VECTOR('',#17390,2.05);
#4547=VECTOR('',#17393,2.05);
#4548=VECTOR('',#17398,3.24999999999999);
#4549=VECTOR('',#17403,10.);
#4550=VECTOR('',#17404,10.);
#4551=VECTOR('',#17405,10.);
#4552=VECTOR('',#17406,10.);
#4553=VECTOR('',#17435,3.05);
#4554=VECTOR('',#17442,3.24999999999999);
#4555=VECTOR('',#17445,3.05);
#4556=VECTOR('',#17452,3.24999999999999);
#4557=VECTOR('',#17455,3.05);
#4558=VECTOR('',#17462,3.25);
#4559=VECTOR('',#17465,3.05);
#4560=VECTOR('',#17472,3.25);
#4561=VECTOR('',#17475,3.05);
#4562=VECTOR('',#17482,3.24999999999999);
#4563=VECTOR('',#17485,3.05);
#4564=VECTOR('',#17490,3.05000000000001);
#4565=VECTOR('',#17493,3.05000000000001);
#4566=VECTOR('',#17496,3.05);
#4567=VECTOR('',#17499,3.05);
#4568=VECTOR('',#17502,3.05);
#4569=VECTOR('',#17505,3.05);
#4570=VECTOR('',#17510,5.65000000000001);
#4571=VECTOR('',#17513,5.50000000000001);
#4572=VECTOR('',#17520,5.65);
#4573=VECTOR('',#17523,5.50000000000001);
#4574=VECTOR('',#17530,5.65);
#4575=VECTOR('',#17533,5.5);
#4576=VECTOR('',#17540,5.65);
#4577=VECTOR('',#17543,5.50000000000001);
#4578=VECTOR('',#17550,5.65);
#4579=VECTOR('',#17553,5.5);
#4580=VECTOR('',#17560,5.65);
#4581=VECTOR('',#17563,5.50000000000001);
#4582=VECTOR('',#17570,5.65);
#4583=VECTOR('',#17573,5.50000000000001);
#4584=VECTOR('',#17580,5.65000000000001);
#4585=VECTOR('',#17583,5.50000000000001);
#4586=VECTOR('',#17620,3.50000000000001);
#4587=VECTOR('',#17625,3.5);
#4588=VECTOR('',#17630,3.5);
#4589=VECTOR('',#17635,3.5);
#4590=VECTOR('',#17640,3.5);
#4591=VECTOR('',#17645,3.5);
#4592=VECTOR('',#17650,3.5);
#4593=VECTOR('',#17655,3.50000000000001);
#4594=VECTOR('',#17660,10.);
#4595=VECTOR('',#17661,10.);
#4596=VECTOR('',#17662,10.);
#4597=VECTOR('',#17665,10.);
#4598=VECTOR('',#17666,10.);
#4599=VECTOR('',#17667,10.);
#4600=VECTOR('',#17670,10.);
#4601=VECTOR('',#17671,10.);
#4602=VECTOR('',#17674,9.99999999999999);
#4603=VECTOR('',#17675,10.);
#4604=VECTOR('',#17676,9.99999999999999);
#4605=VECTOR('',#17679,10.);
#4606=VECTOR('',#17682,10.);
#4607=VECTOR('',#17683,10.);
#4608=VECTOR('',#17686,10.);
#4609=VECTOR('',#17687,10.);
#4610=VECTOR('',#17690,10.);
#4611=VECTOR('',#17695,10.);
#4612=VECTOR('',#17696,10.);
#4613=VECTOR('',#17699,10.);
#4614=VECTOR('',#17702,10.);
#4615=VECTOR('',#17703,10.);
#4616=VECTOR('',#17706,10.);
#4617=VECTOR('',#17713,10.);
#4618=VECTOR('',#17716,10.);
#4619=VECTOR('',#17719,10.);
#4620=VECTOR('',#17722,10.);
#4621=VECTOR('',#17725,10.);
#5492=CIRCLE('',#15329,2.55000000000001);
#5493=CIRCLE('',#15330,2.85);
#5494=CIRCLE('',#15331,2.85);
#5495=CIRCLE('',#15333,5.);
#5496=CIRCLE('',#15334,5.30000000000001);
#5497=CIRCLE('',#15335,5.30000000000001);
#5498=CIRCLE('',#15337,2.55000000000001);
#5499=CIRCLE('',#15339,2.55000000000001);
#5500=CIRCLE('',#15340,2.85);
#5501=CIRCLE('',#15341,2.85);
#5502=CIRCLE('',#15343,5.);
#5503=CIRCLE('',#15344,5.29999999999999);
#5504=CIRCLE('',#15345,5.29999999999999);
#5505=CIRCLE('',#15347,2.55000000000001);
#5506=CIRCLE('',#15349,2.55);
#5507=CIRCLE('',#15350,2.85);
#5508=CIRCLE('',#15351,2.85);
#5509=CIRCLE('',#15353,5.);
#5510=CIRCLE('',#15354,5.3);
#5511=CIRCLE('',#15355,5.3);
#5512=CIRCLE('',#15357,2.55);
#5513=CIRCLE('',#15360,5.);
#5514=CIRCLE('',#15362,5.);
#5515=CIRCLE('',#15364,5.);
#5516=CIRCLE('',#15366,3.);
#5517=CIRCLE('',#15368,3.00000000000001);
#5518=CIRCLE('',#15370,3.00000000000001);
#5519=CIRCLE('',#15372,3.);
#5520=CIRCLE('',#15374,3.00000000000001);
#5521=CIRCLE('',#15376,3.00000000000001);
#5522=CIRCLE('',#15378,2.55000000000001);
#5523=CIRCLE('',#15379,2.85);
#5524=CIRCLE('',#15380,2.85);
#5525=CIRCLE('',#15382,5.);
#5526=CIRCLE('',#15383,5.30000000000001);
#5527=CIRCLE('',#15384,5.30000000000001);
#5528=CIRCLE('',#15386,2.55000000000001);
#5529=CIRCLE('',#15388,2.55000000000001);
#5530=CIRCLE('',#15389,2.85);
#5531=CIRCLE('',#15390,2.85);
#5532=CIRCLE('',#15392,5.);
#5533=CIRCLE('',#15393,5.29999999999999);
#5534=CIRCLE('',#15394,5.29999999999999);
#5535=CIRCLE('',#15396,2.55000000000001);
#5536=CIRCLE('',#15398,2.55);
#5537=CIRCLE('',#15399,2.85);
#5538=CIRCLE('',#15400,2.85);
#5539=CIRCLE('',#15402,5.);
#5540=CIRCLE('',#15403,5.3);
#5541=CIRCLE('',#15404,5.3);
#5542=CIRCLE('',#15406,2.55);
#5543=CIRCLE('',#15409,5.);
#5544=CIRCLE('',#15411,5.);
#5545=CIRCLE('',#15413,5.);
#5546=CIRCLE('',#15415,3.);
#5547=CIRCLE('',#15417,3.00000000000001);
#5548=CIRCLE('',#15419,3.00000000000001);
#5549=CIRCLE('',#15421,3.);
#5550=CIRCLE('',#15423,3.00000000000001);
#5551=CIRCLE('',#15425,3.00000000000001);
#5552=CIRCLE('',#15427,2.05);
#5553=CIRCLE('',#15428,2.34999999999999);
#5554=CIRCLE('',#15430,2.35);
#5555=CIRCLE('',#15431,2.35);
#5556=CIRCLE('',#15432,2.35);
#5557=CIRCLE('',#15434,2.05);
#5558=CIRCLE('',#15435,2.05);
#5559=CIRCLE('',#15437,2.05);
#5560=CIRCLE('',#15439,2.05);
#5561=CIRCLE('',#15440,2.05);
#5562=CIRCLE('',#15442,2.05);
#5563=CIRCLE('',#15444,2.05);
#5564=CIRCLE('',#15445,2.05);
#5565=CIRCLE('',#15447,2.05);
#5566=CIRCLE('',#15449,2.05);
#5567=CIRCLE('',#15450,2.05);
#5568=CIRCLE('',#15456,2.05);
#5569=CIRCLE('',#15457,2.34999999999999);
#5570=CIRCLE('',#15459,2.35);
#5571=CIRCLE('',#15460,2.35);
#5572=CIRCLE('',#15461,2.35);
#5573=CIRCLE('',#15463,2.05);
#5574=CIRCLE('',#15464,2.05);
#5575=CIRCLE('',#15466,2.05);
#5576=CIRCLE('',#15468,2.05);
#5577=CIRCLE('',#15469,2.05);
#5578=CIRCLE('',#15471,2.05);
#5579=CIRCLE('',#15473,2.05);
#5580=CIRCLE('',#15474,2.05);
#5581=CIRCLE('',#15476,2.05);
#5582=CIRCLE('',#15478,2.05);
#5583=CIRCLE('',#15479,2.05);
#5584=CIRCLE('',#15485,3.05);
#5585=CIRCLE('',#15486,3.44999999999999);
#5586=CIRCLE('',#15488,3.44999999999999);
#5587=CIRCLE('',#15489,3.45);
#5588=CIRCLE('',#15490,3.44999999999999);
#5589=CIRCLE('',#15491,5.80000000000002);
#5590=CIRCLE('',#15492,5.8);
#5591=CIRCLE('',#15493,5.8);
#5592=CIRCLE('',#15494,5.8);
#5593=CIRCLE('',#15495,5.80000000000002);
#5594=CIRCLE('',#15496,5.8);
#5595=CIRCLE('',#15497,5.8);
#5596=CIRCLE('',#15498,5.8);
#5597=CIRCLE('',#15499,3.45);
#5598=CIRCLE('',#15500,3.44999999999999);
#5599=CIRCLE('',#15502,3.05);
#5600=CIRCLE('',#15504,3.05);
#5601=CIRCLE('',#15506,3.05);
#5602=CIRCLE('',#15508,3.05);
#5603=CIRCLE('',#15510,3.05);
#5604=CIRCLE('',#15512,3.05);
#5605=CIRCLE('',#15514,3.05);
#5606=CIRCLE('',#15516,3.05);
#5607=CIRCLE('',#15518,3.05);
#5608=CIRCLE('',#15520,3.05);
#5609=CIRCLE('',#15522,3.05);
#5610=CIRCLE('',#15530,5.50000000000001);
#5611=CIRCLE('',#15532,5.50000000000001);
#5612=CIRCLE('',#15534,5.50000000000001);
#5613=CIRCLE('',#15536,5.50000000000001);
#5614=CIRCLE('',#15538,5.5);
#5615=CIRCLE('',#15540,5.5);
#5616=CIRCLE('',#15542,5.50000000000001);
#5617=CIRCLE('',#15544,5.50000000000001);
#5618=CIRCLE('',#15546,5.5);
#5619=CIRCLE('',#15548,5.5);
#5620=CIRCLE('',#15550,5.50000000000001);
#5621=CIRCLE('',#15552,5.50000000000001);
#5622=CIRCLE('',#15554,5.50000000000001);
#5623=CIRCLE('',#15556,5.50000000000001);
#5624=CIRCLE('',#15558,5.50000000000001);
#5625=CIRCLE('',#15560,5.50000000000001);
#5626=CIRCLE('',#15562,3.50000000000001);
#5627=CIRCLE('',#15564,3.5);
#5628=CIRCLE('',#15566,3.5);
#5629=CIRCLE('',#15568,3.5);
#5630=CIRCLE('',#15570,3.5);
#5631=CIRCLE('',#15572,3.5);
#5632=CIRCLE('',#15574,3.5);
#5633=CIRCLE('',#15576,3.50000000000001);
#5634=CIRCLE('',#15578,3.50000000000001);
#5635=CIRCLE('',#15580,3.5);
#5636=CIRCLE('',#15582,3.5);
#5637=CIRCLE('',#15584,3.5);
#5638=CIRCLE('',#15586,3.5);
#5639=CIRCLE('',#15588,3.5);
#5640=CIRCLE('',#15590,3.5);
#5641=CIRCLE('',#15592,3.50000000000001);
#6133=VERTEX_POINT('',#20924);
#6134=VERTEX_POINT('',#20926);
#6135=VERTEX_POINT('',#20928);
#6136=VERTEX_POINT('',#20930);
#6137=VERTEX_POINT('',#20939);
#6138=VERTEX_POINT('',#20941);
#6139=VERTEX_POINT('',#20946);
#6140=VERTEX_POINT('',#20950);
#6141=VERTEX_POINT('',#20952);
#6142=VERTEX_POINT('',#20954);
#6143=VERTEX_POINT('',#20956);
#6144=VERTEX_POINT('',#20965);
#6145=VERTEX_POINT('',#20967);
#6146=VERTEX_POINT('',#20972);
#6147=VERTEX_POINT('',#20976);
#6148=VERTEX_POINT('',#20978);
#6149=VERTEX_POINT('',#20980);
#6150=VERTEX_POINT('',#20982);
#6151=VERTEX_POINT('',#20991);
#6152=VERTEX_POINT('',#20993);
#6153=VERTEX_POINT('',#20998);
#6154=VERTEX_POINT('',#21002);
#6155=VERTEX_POINT('',#21003);
#6156=VERTEX_POINT('',#21005);
#6157=VERTEX_POINT('',#21007);
#6158=VERTEX_POINT('',#21011);
#6159=VERTEX_POINT('',#21015);
#6160=VERTEX_POINT('',#21019);
#6161=VERTEX_POINT('',#21023);
#6162=VERTEX_POINT('',#21026);
#6163=VERTEX_POINT('',#21029);
#6164=VERTEX_POINT('',#21032);
#6165=VERTEX_POINT('',#21036);
#6166=VERTEX_POINT('',#21040);
#6167=VERTEX_POINT('',#21044);
#6168=VERTEX_POINT('',#21046);
#6169=VERTEX_POINT('',#21048);
#6170=VERTEX_POINT('',#21050);
#6171=VERTEX_POINT('',#21059);
#6172=VERTEX_POINT('',#21061);
#6173=VERTEX_POINT('',#21066);
#6174=VERTEX_POINT('',#21070);
#6175=VERTEX_POINT('',#21072);
#6176=VERTEX_POINT('',#21074);
#6177=VERTEX_POINT('',#21076);
#6178=VERTEX_POINT('',#21085);
#6179=VERTEX_POINT('',#21087);
#6180=VERTEX_POINT('',#21092);
#6181=VERTEX_POINT('',#21096);
#6182=VERTEX_POINT('',#21098);
#6183=VERTEX_POINT('',#21100);
#6184=VERTEX_POINT('',#21102);
#6185=VERTEX_POINT('',#21111);
#6186=VERTEX_POINT('',#21113);
#6187=VERTEX_POINT('',#21118);
#6188=VERTEX_POINT('',#21122);
#6189=VERTEX_POINT('',#21123);
#6190=VERTEX_POINT('',#21125);
#6191=VERTEX_POINT('',#21127);
#6192=VERTEX_POINT('',#21131);
#6193=VERTEX_POINT('',#21135);
#6194=VERTEX_POINT('',#21139);
#6195=VERTEX_POINT('',#21143);
#6196=VERTEX_POINT('',#21146);
#6197=VERTEX_POINT('',#21149);
#6198=VERTEX_POINT('',#21152);
#6199=VERTEX_POINT('',#21156);
#6200=VERTEX_POINT('',#21160);
#6201=VERTEX_POINT('',#21164);
#6202=VERTEX_POINT('',#21166);
#6203=VERTEX_POINT('',#21170);
#6204=VERTEX_POINT('',#21171);
#6205=VERTEX_POINT('',#21173);
#6206=VERTEX_POINT('',#21175);
#6207=VERTEX_POINT('',#21177);
#6208=VERTEX_POINT('',#21179);
#6209=VERTEX_POINT('',#21181);
#6210=VERTEX_POINT('',#21183);
#6211=VERTEX_POINT('',#21185);
#6212=VERTEX_POINT('',#21187);
#6213=VERTEX_POINT('',#21189);
#6214=VERTEX_POINT('',#21191);
#6215=VERTEX_POINT('',#21193);
#6216=VERTEX_POINT('',#21195);
#6217=VERTEX_POINT('',#21198);
#6218=VERTEX_POINT('',#21200);
#6219=VERTEX_POINT('',#21202);
#6220=VERTEX_POINT('',#21205);
#6221=VERTEX_POINT('',#21207);
#6222=VERTEX_POINT('',#21211);
#6223=VERTEX_POINT('',#21215);
#6224=VERTEX_POINT('',#21217);
#6225=VERTEX_POINT('',#21221);
#6226=VERTEX_POINT('',#21225);
#6227=VERTEX_POINT('',#21227);
#6228=VERTEX_POINT('',#21231);
#6229=VERTEX_POINT('',#21235);
#6230=VERTEX_POINT('',#21237);
#6231=VERTEX_POINT('',#21241);
#6232=VERTEX_POINT('',#21244);
#6233=VERTEX_POINT('',#21247);
#6234=VERTEX_POINT('',#21250);
#6235=VERTEX_POINT('',#21253);
#6236=VERTEX_POINT('',#21255);
#6237=VERTEX_POINT('',#21259);
#6238=VERTEX_POINT('',#21260);
#6239=VERTEX_POINT('',#21262);
#6240=VERTEX_POINT('',#21264);
#6241=VERTEX_POINT('',#21266);
#6242=VERTEX_POINT('',#21268);
#6243=VERTEX_POINT('',#21270);
#6244=VERTEX_POINT('',#21272);
#6245=VERTEX_POINT('',#21274);
#6246=VERTEX_POINT('',#21276);
#6247=VERTEX_POINT('',#21278);
#6248=VERTEX_POINT('',#21280);
#6249=VERTEX_POINT('',#21282);
#6250=VERTEX_POINT('',#21284);
#6251=VERTEX_POINT('',#21287);
#6252=VERTEX_POINT('',#21289);
#6253=VERTEX_POINT('',#21291);
#6254=VERTEX_POINT('',#21294);
#6255=VERTEX_POINT('',#21296);
#6256=VERTEX_POINT('',#21300);
#6257=VERTEX_POINT('',#21304);
#6258=VERTEX_POINT('',#21306);
#6259=VERTEX_POINT('',#21310);
#6260=VERTEX_POINT('',#21314);
#6261=VERTEX_POINT('',#21316);
#6262=VERTEX_POINT('',#21320);
#6263=VERTEX_POINT('',#21324);
#6264=VERTEX_POINT('',#21326);
#6265=VERTEX_POINT('',#21330);
#6266=VERTEX_POINT('',#21333);
#6267=VERTEX_POINT('',#21336);
#6268=VERTEX_POINT('',#21339);
#6269=VERTEX_POINT('',#21342);
#6270=VERTEX_POINT('',#21344);
#6271=VERTEX_POINT('',#21348);
#6272=VERTEX_POINT('',#21349);
#6273=VERTEX_POINT('',#21351);
#6274=VERTEX_POINT('',#21353);
#6275=VERTEX_POINT('',#21356);
#6276=VERTEX_POINT('',#21358);
#6277=VERTEX_POINT('',#21360);
#6278=VERTEX_POINT('',#21362);
#6279=VERTEX_POINT('',#21364);
#6280=VERTEX_POINT('',#21366);
#6281=VERTEX_POINT('',#21368);
#6282=VERTEX_POINT('',#21370);
#6283=VERTEX_POINT('',#21372);
#6284=VERTEX_POINT('',#21374);
#6285=VERTEX_POINT('',#21376);
#6286=VERTEX_POINT('',#21378);
#6287=VERTEX_POINT('',#21380);
#6288=VERTEX_POINT('',#21383);
#6289=VERTEX_POINT('',#21387);
#6290=VERTEX_POINT('',#21391);
#6291=VERTEX_POINT('',#21395);
#6292=VERTEX_POINT('',#21399);
#6293=VERTEX_POINT('',#21403);
#6294=VERTEX_POINT('',#21407);
#6295=VERTEX_POINT('',#21411);
#6296=VERTEX_POINT('',#21415);
#6297=VERTEX_POINT('',#21419);
#6298=VERTEX_POINT('',#21423);
#6299=VERTEX_POINT('',#21427);
#6300=VERTEX_POINT('',#21430);
#6301=VERTEX_POINT('',#21433);
#6302=VERTEX_POINT('',#21436);
#6303=VERTEX_POINT('',#21439);
#6304=VERTEX_POINT('',#21442);
#6305=VERTEX_POINT('',#21445);
#6306=VERTEX_POINT('',#21449);
#6307=VERTEX_POINT('',#21453);
#6308=VERTEX_POINT('',#21457);
#6309=VERTEX_POINT('',#21461);
#6310=VERTEX_POINT('',#21465);
#6311=VERTEX_POINT('',#21469);
#6312=VERTEX_POINT('',#21473);
#6313=VERTEX_POINT('',#21477);
#6314=VERTEX_POINT('',#21481);
#6315=VERTEX_POINT('',#21485);
#6316=VERTEX_POINT('',#21489);
#6317=VERTEX_POINT('',#21493);
#6318=VERTEX_POINT('',#21497);
#6319=VERTEX_POINT('',#21501);
#6320=VERTEX_POINT('',#21505);
#6321=VERTEX_POINT('',#21509);
#6322=VERTEX_POINT('',#21512);
#6323=VERTEX_POINT('',#21515);
#6324=VERTEX_POINT('',#21518);
#6325=VERTEX_POINT('',#21521);
#6326=VERTEX_POINT('',#21524);
#6327=VERTEX_POINT('',#21527);
#6328=VERTEX_POINT('',#21530);
#6329=VERTEX_POINT('',#21533);
#6330=VERTEX_POINT('',#21537);
#6331=VERTEX_POINT('',#21541);
#6332=VERTEX_POINT('',#21545);
#6333=VERTEX_POINT('',#21549);
#6334=VERTEX_POINT('',#21553);
#6335=VERTEX_POINT('',#21557);
#6336=VERTEX_POINT('',#21561);
#6337=VERTEX_POINT('',#21566);
#6338=VERTEX_POINT('',#21570);
#6339=VERTEX_POINT('',#21579);
#6340=VERTEX_POINT('',#21588);
#7728=EDGE_CURVE('',#6133,#6133,#5492,.T.);
#7729=EDGE_CURVE('',#6133,#6134,#3346,.T.);
#7730=EDGE_CURVE('',#6134,#6135,#5493,.T.);
#7731=EDGE_CURVE('',#6135,#6136,#402,.T.);
#7732=EDGE_CURVE('',#6136,#6134,#5494,.T.);
#7733=EDGE_CURVE('',#6137,#6137,#5495,.T.);
#7734=EDGE_CURVE('',#6137,#6138,#3347,.T.);
#7735=EDGE_CURVE('',#6138,#6136,#5496,.T.);
#7736=EDGE_CURVE('',#6135,#6138,#5497,.T.);
#7737=EDGE_CURVE('',#6133,#6139,#3348,.T.);
#7738=EDGE_CURVE('',#6139,#6139,#5498,.T.);
#7739=EDGE_CURVE('',#6140,#6140,#5499,.T.);
#7740=EDGE_CURVE('',#6140,#6141,#3349,.T.);
#7741=EDGE_CURVE('',#6141,#6142,#5500,.T.);
#7742=EDGE_CURVE('',#6142,#6143,#403,.T.);
#7743=EDGE_CURVE('',#6143,#6141,#5501,.T.);
#7744=EDGE_CURVE('',#6144,#6144,#5502,.T.);
#7745=EDGE_CURVE('',#6144,#6145,#3350,.T.);
#7746=EDGE_CURVE('',#6145,#6143,#5503,.T.);
#7747=EDGE_CURVE('',#6142,#6145,#5504,.T.);
#7748=EDGE_CURVE('',#6140,#6146,#3351,.T.);
#7749=EDGE_CURVE('',#6146,#6146,#5505,.T.);
#7750=EDGE_CURVE('',#6147,#6147,#5506,.T.);
#7751=EDGE_CURVE('',#6147,#6148,#3352,.T.);
#7752=EDGE_CURVE('',#6148,#6149,#5507,.T.);
#7753=EDGE_CURVE('',#6149,#6150,#404,.T.);
#7754=EDGE_CURVE('',#6150,#6148,#5508,.T.);
#7755=EDGE_CURVE('',#6151,#6151,#5509,.T.);
#7756=EDGE_CURVE('',#6151,#6152,#3353,.T.);
#7757=EDGE_CURVE('',#6152,#6150,#5510,.T.);
#7758=EDGE_CURVE('',#6149,#6152,#5511,.T.);
#7759=EDGE_CURVE('',#6147,#6153,#3354,.T.);
#7760=EDGE_CURVE('',#6153,#6153,#5512,.T.);
#7761=EDGE_CURVE('',#6154,#6155,#3355,.T.);
#7762=EDGE_CURVE('',#6156,#6154,#3356,.T.);
#7763=EDGE_CURVE('',#6157,#6156,#3357,.T.);
#7764=EDGE_CURVE('',#6155,#6157,#3358,.T.);
#7765=EDGE_CURVE('',#6137,#6158,#3359,.T.);
#7766=EDGE_CURVE('',#6158,#6158,#5513,.T.);
#7767=EDGE_CURVE('',#6144,#6159,#3360,.T.);
#7768=EDGE_CURVE('',#6159,#6159,#5514,.T.);
#7769=EDGE_CURVE('',#6151,#6160,#3361,.T.);
#7770=EDGE_CURVE('',#6160,#6160,#5515,.T.);
#7771=EDGE_CURVE('',#6161,#6161,#5516,.T.);
#7772=EDGE_CURVE('',#6162,#6162,#5517,.T.);
#7773=EDGE_CURVE('',#6163,#6163,#5518,.T.);
#7774=EDGE_CURVE('',#6161,#6164,#3362,.T.);
#7775=EDGE_CURVE('',#6164,#6164,#5519,.T.);
#7776=EDGE_CURVE('',#6162,#6165,#3363,.T.);
#7777=EDGE_CURVE('',#6165,#6165,#5520,.T.);
#7778=EDGE_CURVE('',#6163,#6166,#3364,.T.);
#7779=EDGE_CURVE('',#6166,#6166,#5521,.T.);
#7780=EDGE_CURVE('',#6167,#6167,#5522,.T.);
#7781=EDGE_CURVE('',#6167,#6168,#3365,.T.);
#7782=EDGE_CURVE('',#6168,#6169,#5523,.T.);
#7783=EDGE_CURVE('',#6169,#6170,#405,.T.);
#7784=EDGE_CURVE('',#6170,#6168,#5524,.T.);
#7785=EDGE_CURVE('',#6171,#6171,#5525,.T.);
#7786=EDGE_CURVE('',#6171,#6172,#3366,.T.);
#7787=EDGE_CURVE('',#6172,#6170,#5526,.T.);
#7788=EDGE_CURVE('',#6169,#6172,#5527,.T.);
#7789=EDGE_CURVE('',#6167,#6173,#3367,.T.);
#7790=EDGE_CURVE('',#6173,#6173,#5528,.T.);
#7791=EDGE_CURVE('',#6174,#6174,#5529,.T.);
#7792=EDGE_CURVE('',#6174,#6175,#3368,.T.);
#7793=EDGE_CURVE('',#6175,#6176,#5530,.T.);
#7794=EDGE_CURVE('',#6176,#6177,#406,.T.);
#7795=EDGE_CURVE('',#6177,#6175,#5531,.T.);
#7796=EDGE_CURVE('',#6178,#6178,#5532,.T.);
#7797=EDGE_CURVE('',#6178,#6179,#3369,.T.);
#7798=EDGE_CURVE('',#6179,#6177,#5533,.T.);
#7799=EDGE_CURVE('',#6176,#6179,#5534,.T.);
#7800=EDGE_CURVE('',#6174,#6180,#3370,.T.);
#7801=EDGE_CURVE('',#6180,#6180,#5535,.T.);
#7802=EDGE_CURVE('',#6181,#6181,#5536,.T.);
#7803=EDGE_CURVE('',#6181,#6182,#3371,.T.);
#7804=EDGE_CURVE('',#6182,#6183,#5537,.T.);
#7805=EDGE_CURVE('',#6183,#6184,#407,.T.);
#7806=EDGE_CURVE('',#6184,#6182,#5538,.T.);
#7807=EDGE_CURVE('',#6185,#6185,#5539,.T.);
#7808=EDGE_CURVE('',#6185,#6186,#3372,.T.);
#7809=EDGE_CURVE('',#6186,#6184,#5540,.T.);
#7810=EDGE_CURVE('',#6183,#6186,#5541,.T.);
#7811=EDGE_CURVE('',#6181,#6187,#3373,.T.);
#7812=EDGE_CURVE('',#6187,#6187,#5542,.T.);
#7813=EDGE_CURVE('',#6188,#6189,#3374,.T.);
#7814=EDGE_CURVE('',#6190,#6188,#3375,.T.);
#7815=EDGE_CURVE('',#6191,#6190,#3376,.T.);
#7816=EDGE_CURVE('',#6189,#6191,#3377,.T.);
#7817=EDGE_CURVE('',#6171,#6192,#3378,.T.);
#7818=EDGE_CURVE('',#6192,#6192,#5543,.T.);
#7819=EDGE_CURVE('',#6178,#6193,#3379,.T.);
#7820=EDGE_CURVE('',#6193,#6193,#5544,.T.);
#7821=EDGE_CURVE('',#6185,#6194,#3380,.T.);
#7822=EDGE_CURVE('',#6194,#6194,#5545,.T.);
#7823=EDGE_CURVE('',#6195,#6195,#5546,.T.);
#7824=EDGE_CURVE('',#6196,#6196,#5547,.T.);
#7825=EDGE_CURVE('',#6197,#6197,#5548,.T.);
#7826=EDGE_CURVE('',#6195,#6198,#3381,.T.);
#7827=EDGE_CURVE('',#6198,#6198,#5549,.T.);
#7828=EDGE_CURVE('',#6196,#6199,#3382,.T.);
#7829=EDGE_CURVE('',#6199,#6199,#5550,.T.);
#7830=EDGE_CURVE('',#6197,#6200,#3383,.T.);
#7831=EDGE_CURVE('',#6200,#6200,#5551,.T.);
#7832=EDGE_CURVE('',#6201,#6201,#5552,.T.);
#7833=EDGE_CURVE('',#6201,#6202,#3384,.T.);
#7834=EDGE_CURVE('',#6202,#6202,#5553,.T.);
#7835=EDGE_CURVE('',#6203,#6204,#3385,.T.);
#7836=EDGE_CURVE('',#6203,#6205,#3386,.T.);
#7837=EDGE_CURVE('',#6206,#6205,#3387,.T.);
#7838=EDGE_CURVE('',#6206,#6207,#3388,.T.);
#7839=EDGE_CURVE('',#6207,#6208,#3389,.T.);
#7840=EDGE_CURVE('',#6208,#6209,#3390,.T.);
#7841=EDGE_CURVE('',#6209,#6210,#3391,.T.);
#7842=EDGE_CURVE('',#6210,#6211,#3392,.T.);
#7843=EDGE_CURVE('',#6211,#6212,#3393,.T.);
#7844=EDGE_CURVE('',#6212,#6213,#3394,.T.);
#7845=EDGE_CURVE('',#6214,#6213,#3395,.T.);
#7846=EDGE_CURVE('',#6214,#6215,#3396,.T.);
#7847=EDGE_CURVE('',#6216,#6215,#3397,.T.);
#7848=EDGE_CURVE('',#6204,#6216,#3398,.T.);
#7849=EDGE_CURVE('',#6217,#6217,#5554,.T.);
#7850=EDGE_CURVE('',#6218,#6218,#5555,.T.);
#7851=EDGE_CURVE('',#6219,#6219,#5556,.T.);
#7852=EDGE_CURVE('',#6201,#6220,#3399,.T.);
#7853=EDGE_CURVE('',#6220,#6221,#5557,.T.);
#7854=EDGE_CURVE('',#6221,#6220,#5558,.T.);
#7855=EDGE_CURVE('',#6222,#6222,#5559,.T.);
#7856=EDGE_CURVE('',#6222,#6217,#3400,.T.);
#7857=EDGE_CURVE('',#6222,#6223,#3401,.T.);
#7858=EDGE_CURVE('',#6223,#6224,#5560,.T.);
#7859=EDGE_CURVE('',#6224,#6223,#5561,.T.);
#7860=EDGE_CURVE('',#6225,#6225,#5562,.T.);
#7861=EDGE_CURVE('',#6225,#6219,#3402,.T.);
#7862=EDGE_CURVE('',#6225,#6226,#3403,.T.);
#7863=EDGE_CURVE('',#6226,#6227,#5563,.T.);
#7864=EDGE_CURVE('',#6227,#6226,#5564,.T.);
#7865=EDGE_CURVE('',#6228,#6228,#5565,.T.);
#7866=EDGE_CURVE('',#6228,#6218,#3404,.T.);
#7867=EDGE_CURVE('',#6228,#6229,#3405,.T.);
#7868=EDGE_CURVE('',#6229,#6230,#5566,.T.);
#7869=EDGE_CURVE('',#6230,#6229,#5567,.T.);
#7870=EDGE_CURVE('',#6231,#6221,#3406,.T.);
#7871=EDGE_CURVE('',#6232,#6230,#3407,.T.);
#7872=EDGE_CURVE('',#6233,#6227,#3408,.T.);
#7873=EDGE_CURVE('',#6234,#6224,#3409,.T.);
#7874=EDGE_CURVE('',#6235,#6235,#5568,.T.);
#7875=EDGE_CURVE('',#6235,#6236,#3410,.T.);
#7876=EDGE_CURVE('',#6236,#6236,#5569,.T.);
#7877=EDGE_CURVE('',#6237,#6238,#3411,.T.);
#7878=EDGE_CURVE('',#6239,#6237,#3412,.T.);
#7879=EDGE_CURVE('',#6240,#6239,#3413,.T.);
#7880=EDGE_CURVE('',#6241,#6240,#3414,.T.);
#7881=EDGE_CURVE('',#6242,#6241,#3415,.T.);
#7882=EDGE_CURVE('',#6243,#6242,#3416,.T.);
#7883=EDGE_CURVE('',#6244,#6243,#3417,.T.);
#7884=EDGE_CURVE('',#6245,#6244,#3418,.T.);
#7885=EDGE_CURVE('',#6246,#6245,#3419,.T.);
#7886=EDGE_CURVE('',#6247,#6246,#3420,.T.);
#7887=EDGE_CURVE('',#6248,#6247,#3421,.T.);
#7888=EDGE_CURVE('',#6249,#6248,#3422,.T.);
#7889=EDGE_CURVE('',#6250,#6249,#3423,.T.);
#7890=EDGE_CURVE('',#6238,#6250,#3424,.T.);
#7891=EDGE_CURVE('',#6251,#6251,#5570,.T.);
#7892=EDGE_CURVE('',#6252,#6252,#5571,.T.);
#7893=EDGE_CURVE('',#6253,#6253,#5572,.T.);
#7894=EDGE_CURVE('',#6235,#6254,#3425,.T.);
#7895=EDGE_CURVE('',#6254,#6255,#5573,.T.);
#7896=EDGE_CURVE('',#6255,#6254,#5574,.T.);
#7897=EDGE_CURVE('',#6256,#6256,#5575,.T.);
#7898=EDGE_CURVE('',#6256,#6251,#3426,.T.);
#7899=EDGE_CURVE('',#6256,#6257,#3427,.T.);
#7900=EDGE_CURVE('',#6257,#6258,#5576,.T.);
#7901=EDGE_CURVE('',#6258,#6257,#5577,.T.);
#7902=EDGE_CURVE('',#6259,#6259,#5578,.T.);
#7903=EDGE_CURVE('',#6259,#6253,#3428,.T.);
#7904=EDGE_CURVE('',#6259,#6260,#3429,.T.);
#7905=EDGE_CURVE('',#6260,#6261,#5579,.T.);
#7906=EDGE_CURVE('',#6261,#6260,#5580,.T.);
#7907=EDGE_CURVE('',#6262,#6262,#5581,.T.);
#7908=EDGE_CURVE('',#6262,#6252,#3430,.T.);
#7909=EDGE_CURVE('',#6262,#6263,#3431,.T.);
#7910=EDGE_CURVE('',#6263,#6264,#5582,.T.);
#7911=EDGE_CURVE('',#6264,#6263,#5583,.T.);
#7912=EDGE_CURVE('',#6265,#6255,#3432,.T.);
#7913=EDGE_CURVE('',#6266,#6264,#3433,.T.);
#7914=EDGE_CURVE('',#6267,#6261,#3434,.T.);
#7915=EDGE_CURVE('',#6268,#6258,#3435,.T.);
#7916=EDGE_CURVE('',#6269,#6269,#5584,.T.);
#7917=EDGE_CURVE('',#6269,#6270,#3436,.T.);
#7918=EDGE_CURVE('',#6270,#6270,#5585,.T.);
#7919=EDGE_CURVE('',#6271,#6272,#3437,.T.);
#7920=EDGE_CURVE('',#6273,#6271,#3438,.T.);
#7921=EDGE_CURVE('',#6274,#6273,#3439,.T.);
#7922=EDGE_CURVE('',#6272,#6274,#3440,.T.);
#7923=EDGE_CURVE('',#6275,#6275,#5586,.T.);
#7924=EDGE_CURVE('',#6276,#6276,#5587,.T.);
#7925=EDGE_CURVE('',#6277,#6277,#5588,.T.);
#7926=EDGE_CURVE('',#6278,#6278,#5589,.T.);
#7927=EDGE_CURVE('',#6279,#6279,#5590,.T.);
#7928=EDGE_CURVE('',#6280,#6280,#5591,.T.);
#7929=EDGE_CURVE('',#6281,#6281,#5592,.T.);
#7930=EDGE_CURVE('',#6282,#6282,#5593,.T.);
#7931=EDGE_CURVE('',#6283,#6283,#5594,.T.);
#7932=EDGE_CURVE('',#6284,#6284,#5595,.T.);
#7933=EDGE_CURVE('',#6285,#6285,#5596,.T.);
#7934=EDGE_CURVE('',#6286,#6286,#5597,.T.);
#7935=EDGE_CURVE('',#6287,#6287,#5598,.T.);
#7936=EDGE_CURVE('',#6269,#6288,#3441,.T.);
#7937=EDGE_CURVE('',#6288,#6288,#5599,.T.);
#7938=EDGE_CURVE('',#6289,#6289,#5600,.T.);
#7939=EDGE_CURVE('',#6289,#6275,#3442,.T.);
#7940=EDGE_CURVE('',#6289,#6290,#3443,.T.);
#7941=EDGE_CURVE('',#6290,#6290,#5601,.T.);
#7942=EDGE_CURVE('',#6291,#6291,#5602,.T.);
#7943=EDGE_CURVE('',#6291,#6287,#3444,.T.);
#7944=EDGE_CURVE('',#6291,#6292,#3445,.T.);
#7945=EDGE_CURVE('',#6292,#6292,#5603,.T.);
#7946=EDGE_CURVE('',#6293,#6293,#5604,.T.);
#7947=EDGE_CURVE('',#6293,#6276,#3446,.T.);
#7948=EDGE_CURVE('',#6293,#6294,#3447,.T.);
#7949=EDGE_CURVE('',#6294,#6294,#5605,.T.);
#7950=EDGE_CURVE('',#6295,#6295,#5606,.T.);
#7951=EDGE_CURVE('',#6295,#6286,#3448,.T.);
#7952=EDGE_CURVE('',#6295,#6296,#3449,.T.);
#7953=EDGE_CURVE('',#6296,#6296,#5607,.T.);
#7954=EDGE_CURVE('',#6297,#6297,#5608,.T.);
#7955=EDGE_CURVE('',#6297,#6277,#3450,.T.);
#7956=EDGE_CURVE('',#6297,#6298,#3451,.T.);
#7957=EDGE_CURVE('',#6298,#6298,#5609,.T.);
#7958=EDGE_CURVE('',#6299,#6288,#3452,.T.);
#7959=EDGE_CURVE('',#6300,#6298,#3453,.T.);
#7960=EDGE_CURVE('',#6301,#6290,#3454,.T.);
#7961=EDGE_CURVE('',#6302,#6292,#3455,.T.);
#7962=EDGE_CURVE('',#6303,#6294,#3456,.T.);
#7963=EDGE_CURVE('',#6304,#6296,#3457,.T.);
#7964=EDGE_CURVE('',#6305,#6305,#5610,.T.);
#7965=EDGE_CURVE('',#6305,#6278,#3458,.T.);
#7966=EDGE_CURVE('',#6305,#6306,#3459,.T.);
#7967=EDGE_CURVE('',#6306,#6306,#5611,.T.);
#7968=EDGE_CURVE('',#6307,#6307,#5612,.T.);
#7969=EDGE_CURVE('',#6307,#6285,#3460,.T.);
#7970=EDGE_CURVE('',#6307,#6308,#3461,.T.);
#7971=EDGE_CURVE('',#6308,#6308,#5613,.T.);
#7972=EDGE_CURVE('',#6309,#6309,#5614,.T.);
#7973=EDGE_CURVE('',#6309,#6279,#3462,.T.);
#7974=EDGE_CURVE('',#6309,#6310,#3463,.T.);
#7975=EDGE_CURVE('',#6310,#6310,#5615,.T.);
#7976=EDGE_CURVE('',#6311,#6311,#5616,.T.);
#7977=EDGE_CURVE('',#6311,#6284,#3464,.T.);
#7978=EDGE_CURVE('',#6311,#6312,#3465,.T.);
#7979=EDGE_CURVE('',#6312,#6312,#5617,.T.);
#7980=EDGE_CURVE('',#6313,#6313,#5618,.T.);
#7981=EDGE_CURVE('',#6313,#6280,#3466,.T.);
#7982=EDGE_CURVE('',#6313,#6314,#3467,.T.);
#7983=EDGE_CURVE('',#6314,#6314,#5619,.T.);
#7984=EDGE_CURVE('',#6315,#6315,#5620,.T.);
#7985=EDGE_CURVE('',#6315,#6283,#3468,.T.);
#7986=EDGE_CURVE('',#6315,#6316,#3469,.T.);
#7987=EDGE_CURVE('',#6316,#6316,#5621,.T.);
#7988=EDGE_CURVE('',#6317,#6317,#5622,.T.);
#7989=EDGE_CURVE('',#6317,#6281,#3470,.T.);
#7990=EDGE_CURVE('',#6317,#6318,#3471,.T.);
#7991=EDGE_CURVE('',#6318,#6318,#5623,.T.);
#7992=EDGE_CURVE('',#6319,#6319,#5624,.T.);
#7993=EDGE_CURVE('',#6319,#6282,#3472,.T.);
#7994=EDGE_CURVE('',#6319,#6320,#3473,.T.);
#7995=EDGE_CURVE('',#6320,#6320,#5625,.T.);
#7996=EDGE_CURVE('',#6321,#6321,#5626,.T.);
#7997=EDGE_CURVE('',#6322,#6322,#5627,.T.);
#7998=EDGE_CURVE('',#6323,#6323,#5628,.T.);
#7999=EDGE_CURVE('',#6324,#6324,#5629,.T.);
#8000=EDGE_CURVE('',#6325,#6325,#5630,.T.);
#8001=EDGE_CURVE('',#6326,#6326,#5631,.T.);
#8002=EDGE_CURVE('',#6327,#6327,#5632,.T.);
#8003=EDGE_CURVE('',#6328,#6328,#5633,.T.);
#8004=EDGE_CURVE('',#6321,#6329,#3474,.T.);
#8005=EDGE_CURVE('',#6329,#6329,#5634,.T.);
#8006=EDGE_CURVE('',#6322,#6330,#3475,.T.);
#8007=EDGE_CURVE('',#6330,#6330,#5635,.T.);
#8008=EDGE_CURVE('',#6323,#6331,#3476,.T.);
#8009=EDGE_CURVE('',#6331,#6331,#5636,.T.);
#8010=EDGE_CURVE('',#6324,#6332,#3477,.T.);
#8011=EDGE_CURVE('',#6332,#6332,#5637,.T.);
#8012=EDGE_CURVE('',#6325,#6333,#3478,.T.);
#8013=EDGE_CURVE('',#6333,#6333,#5638,.T.);
#8014=EDGE_CURVE('',#6326,#6334,#3479,.T.);
#8015=EDGE_CURVE('',#6334,#6334,#5639,.T.);
#8016=EDGE_CURVE('',#6327,#6335,#3480,.T.);
#8017=EDGE_CURVE('',#6335,#6335,#5640,.T.);
#8018=EDGE_CURVE('',#6328,#6336,#3481,.T.);
#8019=EDGE_CURVE('',#6336,#6336,#5641,.T.);
#8020=EDGE_CURVE('',#6155,#6203,#3482,.T.);
#8021=EDGE_CURVE('',#6204,#6337,#3483,.T.);
#8022=EDGE_CURVE('',#6337,#6154,#3484,.T.);
#8023=EDGE_CURVE('',#6216,#6338,#3485,.T.);
#8024=EDGE_CURVE('',#6338,#6271,#3486,.T.);
#8025=EDGE_CURVE('',#6272,#6337,#3487,.T.);
#8026=EDGE_CURVE('',#6249,#6157,#3488,.T.);
#8027=EDGE_CURVE('',#6249,#6203,#3489,.T.);
#8028=EDGE_CURVE('',#6189,#6338,#3490,.T.);
#8029=EDGE_CURVE('',#6339,#6191,#3491,.T.);
#8030=EDGE_CURVE('',#6273,#6339,#3492,.T.);
#8031=EDGE_CURVE('',#6215,#6188,#3493,.T.);
#8032=EDGE_CURVE('',#6190,#6237,#3494,.T.);
#8033=EDGE_CURVE('',#6238,#6339,#3495,.T.);
#8034=EDGE_CURVE('',#6250,#6340,#3496,.T.);
#8035=EDGE_CURVE('',#6340,#6274,#3497,.T.);
#8036=EDGE_CURVE('',#6156,#6340,#3498,.T.);
#8037=EDGE_CURVE('',#6213,#6240,#3499,.T.);
#8038=EDGE_CURVE('',#6239,#6214,#3500,.T.);
#8039=EDGE_CURVE('',#6215,#6237,#3501,.T.);
#8040=EDGE_CURVE('',#6205,#6248,#3502,.T.);
#8041=EDGE_CURVE('',#6247,#6206,#3503,.T.);
#8042=EDGE_CURVE('',#6246,#6207,#3504,.T.);
#8043=EDGE_CURVE('',#6241,#6212,#3505,.T.);
#8044=EDGE_CURVE('',#6242,#6211,#3506,.T.);
#8045=EDGE_CURVE('',#6243,#6210,#3507,.T.);
#8046=EDGE_CURVE('',#6244,#6209,#3508,.T.);
#8047=EDGE_CURVE('',#6245,#6208,#3509,.T.);
#10130=ORIENTED_EDGE('',*,*,#7728,.T.);
#10131=ORIENTED_EDGE('',*,*,#7729,.T.);
#10132=ORIENTED_EDGE('',*,*,#7730,.T.);
#10133=ORIENTED_EDGE('',*,*,#7731,.T.);
#10134=ORIENTED_EDGE('',*,*,#7732,.T.);
#10135=ORIENTED_EDGE('',*,*,#7729,.F.);
#10136=ORIENTED_EDGE('',*,*,#7733,.T.);
#10137=ORIENTED_EDGE('',*,*,#7734,.T.);
#10138=ORIENTED_EDGE('',*,*,#7735,.T.);
#10139=ORIENTED_EDGE('',*,*,#7731,.F.);
#10140=ORIENTED_EDGE('',*,*,#7736,.T.);
#10141=ORIENTED_EDGE('',*,*,#7734,.F.);
#10142=ORIENTED_EDGE('',*,*,#7728,.F.);
#10143=ORIENTED_EDGE('',*,*,#7737,.T.);
#10144=ORIENTED_EDGE('',*,*,#7738,.F.);
#10145=ORIENTED_EDGE('',*,*,#7737,.F.);
#10146=ORIENTED_EDGE('',*,*,#7739,.T.);
#10147=ORIENTED_EDGE('',*,*,#7740,.T.);
#10148=ORIENTED_EDGE('',*,*,#7741,.T.);
#10149=ORIENTED_EDGE('',*,*,#7742,.T.);
#10150=ORIENTED_EDGE('',*,*,#7743,.T.);
#10151=ORIENTED_EDGE('',*,*,#7740,.F.);
#10152=ORIENTED_EDGE('',*,*,#7744,.T.);
#10153=ORIENTED_EDGE('',*,*,#7745,.T.);
#10154=ORIENTED_EDGE('',*,*,#7746,.T.);
#10155=ORIENTED_EDGE('',*,*,#7742,.F.);
#10156=ORIENTED_EDGE('',*,*,#7747,.T.);
#10157=ORIENTED_EDGE('',*,*,#7745,.F.);
#10158=ORIENTED_EDGE('',*,*,#7739,.F.);
#10159=ORIENTED_EDGE('',*,*,#7748,.T.);
#10160=ORIENTED_EDGE('',*,*,#7749,.F.);
#10161=ORIENTED_EDGE('',*,*,#7748,.F.);
#10162=ORIENTED_EDGE('',*,*,#7750,.T.);
#10163=ORIENTED_EDGE('',*,*,#7751,.T.);
#10164=ORIENTED_EDGE('',*,*,#7752,.T.);
#10165=ORIENTED_EDGE('',*,*,#7753,.T.);
#10166=ORIENTED_EDGE('',*,*,#7754,.T.);
#10167=ORIENTED_EDGE('',*,*,#7751,.F.);
#10168=ORIENTED_EDGE('',*,*,#7755,.T.);
#10169=ORIENTED_EDGE('',*,*,#7756,.T.);
#10170=ORIENTED_EDGE('',*,*,#7757,.T.);
#10171=ORIENTED_EDGE('',*,*,#7753,.F.);
#10172=ORIENTED_EDGE('',*,*,#7758,.T.);
#10173=ORIENTED_EDGE('',*,*,#7756,.F.);
#10174=ORIENTED_EDGE('',*,*,#7750,.F.);
#10175=ORIENTED_EDGE('',*,*,#7759,.T.);
#10176=ORIENTED_EDGE('',*,*,#7760,.F.);
#10177=ORIENTED_EDGE('',*,*,#7759,.F.);
#10178=ORIENTED_EDGE('',*,*,#7761,.F.);
#10179=ORIENTED_EDGE('',*,*,#7762,.F.);
#10180=ORIENTED_EDGE('',*,*,#7763,.F.);
#10181=ORIENTED_EDGE('',*,*,#7764,.F.);
#10182=ORIENTED_EDGE('',*,*,#7732,.F.);
#10183=ORIENTED_EDGE('',*,*,#7735,.F.);
#10184=ORIENTED_EDGE('',*,*,#7736,.F.);
#10185=ORIENTED_EDGE('',*,*,#7730,.F.);
#10186=ORIENTED_EDGE('',*,*,#7743,.F.);
#10187=ORIENTED_EDGE('',*,*,#7746,.F.);
#10188=ORIENTED_EDGE('',*,*,#7747,.F.);
#10189=ORIENTED_EDGE('',*,*,#7741,.F.);
#10190=ORIENTED_EDGE('',*,*,#7754,.F.);
#10191=ORIENTED_EDGE('',*,*,#7757,.F.);
#10192=ORIENTED_EDGE('',*,*,#7758,.F.);
#10193=ORIENTED_EDGE('',*,*,#7752,.F.);
#10194=ORIENTED_EDGE('',*,*,#7733,.F.);
#10195=ORIENTED_EDGE('',*,*,#7765,.T.);
#10196=ORIENTED_EDGE('',*,*,#7766,.T.);
#10197=ORIENTED_EDGE('',*,*,#7765,.F.);
#10198=ORIENTED_EDGE('',*,*,#7744,.F.);
#10199=ORIENTED_EDGE('',*,*,#7767,.T.);
#10200=ORIENTED_EDGE('',*,*,#7768,.T.);
#10201=ORIENTED_EDGE('',*,*,#7767,.F.);
#10202=ORIENTED_EDGE('',*,*,#7755,.F.);
#10203=ORIENTED_EDGE('',*,*,#7769,.T.);
#10204=ORIENTED_EDGE('',*,*,#7770,.T.);
#10205=ORIENTED_EDGE('',*,*,#7769,.F.);
#10206=ORIENTED_EDGE('',*,*,#7770,.F.);
#10207=ORIENTED_EDGE('',*,*,#7771,.F.);
#10208=ORIENTED_EDGE('',*,*,#7768,.F.);
#10209=ORIENTED_EDGE('',*,*,#7772,.F.);
#10210=ORIENTED_EDGE('',*,*,#7766,.F.);
#10211=ORIENTED_EDGE('',*,*,#7773,.F.);
#10212=ORIENTED_EDGE('',*,*,#7771,.T.);
#10213=ORIENTED_EDGE('',*,*,#7774,.T.);
#10214=ORIENTED_EDGE('',*,*,#7775,.F.);
#10215=ORIENTED_EDGE('',*,*,#7774,.F.);
#10216=ORIENTED_EDGE('',*,*,#7772,.T.);
#10217=ORIENTED_EDGE('',*,*,#7776,.T.);
#10218=ORIENTED_EDGE('',*,*,#7777,.F.);
#10219=ORIENTED_EDGE('',*,*,#7776,.F.);
#10220=ORIENTED_EDGE('',*,*,#7773,.T.);
#10221=ORIENTED_EDGE('',*,*,#7778,.T.);
#10222=ORIENTED_EDGE('',*,*,#7779,.F.);
#10223=ORIENTED_EDGE('',*,*,#7778,.F.);
#10224=ORIENTED_EDGE('',*,*,#7780,.T.);
#10225=ORIENTED_EDGE('',*,*,#7781,.T.);
#10226=ORIENTED_EDGE('',*,*,#7782,.T.);
#10227=ORIENTED_EDGE('',*,*,#7783,.T.);
#10228=ORIENTED_EDGE('',*,*,#7784,.T.);
#10229=ORIENTED_EDGE('',*,*,#7781,.F.);
#10230=ORIENTED_EDGE('',*,*,#7785,.T.);
#10231=ORIENTED_EDGE('',*,*,#7786,.T.);
#10232=ORIENTED_EDGE('',*,*,#7787,.T.);
#10233=ORIENTED_EDGE('',*,*,#7783,.F.);
#10234=ORIENTED_EDGE('',*,*,#7788,.T.);
#10235=ORIENTED_EDGE('',*,*,#7786,.F.);
#10236=ORIENTED_EDGE('',*,*,#7780,.F.);
#10237=ORIENTED_EDGE('',*,*,#7789,.T.);
#10238=ORIENTED_EDGE('',*,*,#7790,.F.);
#10239=ORIENTED_EDGE('',*,*,#7789,.F.);
#10240=ORIENTED_EDGE('',*,*,#7791,.T.);
#10241=ORIENTED_EDGE('',*,*,#7792,.T.);
#10242=ORIENTED_EDGE('',*,*,#7793,.T.);
#10243=ORIENTED_EDGE('',*,*,#7794,.T.);
#10244=ORIENTED_EDGE('',*,*,#7795,.T.);
#10245=ORIENTED_EDGE('',*,*,#7792,.F.);
#10246=ORIENTED_EDGE('',*,*,#7796,.T.);
#10247=ORIENTED_EDGE('',*,*,#7797,.T.);
#10248=ORIENTED_EDGE('',*,*,#7798,.T.);
#10249=ORIENTED_EDGE('',*,*,#7794,.F.);
#10250=ORIENTED_EDGE('',*,*,#7799,.T.);
#10251=ORIENTED_EDGE('',*,*,#7797,.F.);
#10252=ORIENTED_EDGE('',*,*,#7791,.F.);
#10253=ORIENTED_EDGE('',*,*,#7800,.T.);
#10254=ORIENTED_EDGE('',*,*,#7801,.F.);
#10255=ORIENTED_EDGE('',*,*,#7800,.F.);
#10256=ORIENTED_EDGE('',*,*,#7802,.T.);
#10257=ORIENTED_EDGE('',*,*,#7803,.T.);
#10258=ORIENTED_EDGE('',*,*,#7804,.T.);
#10259=ORIENTED_EDGE('',*,*,#7805,.T.);
#10260=ORIENTED_EDGE('',*,*,#7806,.T.);
#10261=ORIENTED_EDGE('',*,*,#7803,.F.);
#10262=ORIENTED_EDGE('',*,*,#7807,.T.);
#10263=ORIENTED_EDGE('',*,*,#7808,.T.);
#10264=ORIENTED_EDGE('',*,*,#7809,.T.);
#10265=ORIENTED_EDGE('',*,*,#7805,.F.);
#10266=ORIENTED_EDGE('',*,*,#7810,.T.);
#10267=ORIENTED_EDGE('',*,*,#7808,.F.);
#10268=ORIENTED_EDGE('',*,*,#7802,.F.);
#10269=ORIENTED_EDGE('',*,*,#7811,.T.);
#10270=ORIENTED_EDGE('',*,*,#7812,.F.);
#10271=ORIENTED_EDGE('',*,*,#7811,.F.);
#10272=ORIENTED_EDGE('',*,*,#7813,.F.);
#10273=ORIENTED_EDGE('',*,*,#7814,.F.);
#10274=ORIENTED_EDGE('',*,*,#7815,.F.);
#10275=ORIENTED_EDGE('',*,*,#7816,.F.);
#10276=ORIENTED_EDGE('',*,*,#7784,.F.);
#10277=ORIENTED_EDGE('',*,*,#7787,.F.);
#10278=ORIENTED_EDGE('',*,*,#7788,.F.);
#10279=ORIENTED_EDGE('',*,*,#7782,.F.);
#10280=ORIENTED_EDGE('',*,*,#7795,.F.);
#10281=ORIENTED_EDGE('',*,*,#7798,.F.);
#10282=ORIENTED_EDGE('',*,*,#7799,.F.);
#10283=ORIENTED_EDGE('',*,*,#7793,.F.);
#10284=ORIENTED_EDGE('',*,*,#7806,.F.);
#10285=ORIENTED_EDGE('',*,*,#7809,.F.);
#10286=ORIENTED_EDGE('',*,*,#7810,.F.);
#10287=ORIENTED_EDGE('',*,*,#7804,.F.);
#10288=ORIENTED_EDGE('',*,*,#7785,.F.);
#10289=ORIENTED_EDGE('',*,*,#7817,.T.);
#10290=ORIENTED_EDGE('',*,*,#7818,.T.);
#10291=ORIENTED_EDGE('',*,*,#7817,.F.);
#10292=ORIENTED_EDGE('',*,*,#7796,.F.);
#10293=ORIENTED_EDGE('',*,*,#7819,.T.);
#10294=ORIENTED_EDGE('',*,*,#7820,.T.);
#10295=ORIENTED_EDGE('',*,*,#7819,.F.);
#10296=ORIENTED_EDGE('',*,*,#7807,.F.);
#10297=ORIENTED_EDGE('',*,*,#7821,.T.);
#10298=ORIENTED_EDGE('',*,*,#7822,.T.);
#10299=ORIENTED_EDGE('',*,*,#7821,.F.);
#10300=ORIENTED_EDGE('',*,*,#7822,.F.);
#10301=ORIENTED_EDGE('',*,*,#7823,.F.);
#10302=ORIENTED_EDGE('',*,*,#7820,.F.);
#10303=ORIENTED_EDGE('',*,*,#7824,.F.);
#10304=ORIENTED_EDGE('',*,*,#7818,.F.);
#10305=ORIENTED_EDGE('',*,*,#7825,.F.);
#10306=ORIENTED_EDGE('',*,*,#7823,.T.);
#10307=ORIENTED_EDGE('',*,*,#7826,.T.);
#10308=ORIENTED_EDGE('',*,*,#7827,.F.);
#10309=ORIENTED_EDGE('',*,*,#7826,.F.);
#10310=ORIENTED_EDGE('',*,*,#7824,.T.);
#10311=ORIENTED_EDGE('',*,*,#7828,.T.);
#10312=ORIENTED_EDGE('',*,*,#7829,.F.);
#10313=ORIENTED_EDGE('',*,*,#7828,.F.);
#10314=ORIENTED_EDGE('',*,*,#7825,.T.);
#10315=ORIENTED_EDGE('',*,*,#7830,.T.);
#10316=ORIENTED_EDGE('',*,*,#7831,.F.);
#10317=ORIENTED_EDGE('',*,*,#7830,.F.);
#10318=ORIENTED_EDGE('',*,*,#7832,.T.);
#10319=ORIENTED_EDGE('',*,*,#7833,.T.);
#10320=ORIENTED_EDGE('',*,*,#7834,.T.);
#10321=ORIENTED_EDGE('',*,*,#7833,.F.);
#10322=ORIENTED_EDGE('',*,*,#7835,.F.);
#10323=ORIENTED_EDGE('',*,*,#7836,.T.);
#10324=ORIENTED_EDGE('',*,*,#7837,.F.);
#10325=ORIENTED_EDGE('',*,*,#7838,.T.);
#10326=ORIENTED_EDGE('',*,*,#7839,.T.);
#10327=ORIENTED_EDGE('',*,*,#7840,.T.);
#10328=ORIENTED_EDGE('',*,*,#7841,.T.);
#10329=ORIENTED_EDGE('',*,*,#7842,.T.);
#10330=ORIENTED_EDGE('',*,*,#7843,.T.);
#10331=ORIENTED_EDGE('',*,*,#7844,.T.);
#10332=ORIENTED_EDGE('',*,*,#7845,.F.);
#10333=ORIENTED_EDGE('',*,*,#7846,.T.);
#10334=ORIENTED_EDGE('',*,*,#7847,.F.);
#10335=ORIENTED_EDGE('',*,*,#7848,.F.);
#10336=ORIENTED_EDGE('',*,*,#7849,.F.);
#10337=ORIENTED_EDGE('',*,*,#7850,.F.);
#10338=ORIENTED_EDGE('',*,*,#7851,.F.);
#10339=ORIENTED_EDGE('',*,*,#7834,.F.);
#10340=ORIENTED_EDGE('',*,*,#7832,.F.);
#10341=ORIENTED_EDGE('',*,*,#7852,.T.);
#10342=ORIENTED_EDGE('',*,*,#7853,.T.);
#10343=ORIENTED_EDGE('',*,*,#7854,.T.);
#10344=ORIENTED_EDGE('',*,*,#7852,.F.);
#10345=ORIENTED_EDGE('',*,*,#7855,.T.);
#10346=ORIENTED_EDGE('',*,*,#7856,.T.);
#10347=ORIENTED_EDGE('',*,*,#7849,.T.);
#10348=ORIENTED_EDGE('',*,*,#7856,.F.);
#10349=ORIENTED_EDGE('',*,*,#7855,.F.);
#10350=ORIENTED_EDGE('',*,*,#7857,.T.);
#10351=ORIENTED_EDGE('',*,*,#7858,.T.);
#10352=ORIENTED_EDGE('',*,*,#7859,.T.);
#10353=ORIENTED_EDGE('',*,*,#7857,.F.);
#10354=ORIENTED_EDGE('',*,*,#7860,.T.);
#10355=ORIENTED_EDGE('',*,*,#7861,.T.);
#10356=ORIENTED_EDGE('',*,*,#7851,.T.);
#10357=ORIENTED_EDGE('',*,*,#7861,.F.);
#10358=ORIENTED_EDGE('',*,*,#7860,.F.);
#10359=ORIENTED_EDGE('',*,*,#7862,.T.);
#10360=ORIENTED_EDGE('',*,*,#7863,.T.);
#10361=ORIENTED_EDGE('',*,*,#7864,.T.);
#10362=ORIENTED_EDGE('',*,*,#7862,.F.);
#10363=ORIENTED_EDGE('',*,*,#7865,.T.);
#10364=ORIENTED_EDGE('',*,*,#7866,.T.);
#10365=ORIENTED_EDGE('',*,*,#7850,.T.);
#10366=ORIENTED_EDGE('',*,*,#7866,.F.);
#10367=ORIENTED_EDGE('',*,*,#7865,.F.);
#10368=ORIENTED_EDGE('',*,*,#7867,.T.);
#10369=ORIENTED_EDGE('',*,*,#7868,.T.);
#10370=ORIENTED_EDGE('',*,*,#7869,.T.);
#10371=ORIENTED_EDGE('',*,*,#7867,.F.);
#10372=ORIENTED_EDGE('',*,*,#7870,.T.);
#10373=ORIENTED_EDGE('',*,*,#7853,.F.);
#10374=ORIENTED_EDGE('',*,*,#7854,.F.);
#10375=ORIENTED_EDGE('',*,*,#7870,.F.);
#10376=ORIENTED_EDGE('',*,*,#7871,.T.);
#10377=ORIENTED_EDGE('',*,*,#7868,.F.);
#10378=ORIENTED_EDGE('',*,*,#7869,.F.);
#10379=ORIENTED_EDGE('',*,*,#7871,.F.);
#10380=ORIENTED_EDGE('',*,*,#7872,.T.);
#10381=ORIENTED_EDGE('',*,*,#7863,.F.);
#10382=ORIENTED_EDGE('',*,*,#7864,.F.);
#10383=ORIENTED_EDGE('',*,*,#7872,.F.);
#10384=ORIENTED_EDGE('',*,*,#7873,.T.);
#10385=ORIENTED_EDGE('',*,*,#7858,.F.);
#10386=ORIENTED_EDGE('',*,*,#7859,.F.);
#10387=ORIENTED_EDGE('',*,*,#7873,.F.);
#10388=ORIENTED_EDGE('',*,*,#7874,.T.);
#10389=ORIENTED_EDGE('',*,*,#7875,.T.);
#10390=ORIENTED_EDGE('',*,*,#7876,.T.);
#10391=ORIENTED_EDGE('',*,*,#7875,.F.);
#10392=ORIENTED_EDGE('',*,*,#7877,.F.);
#10393=ORIENTED_EDGE('',*,*,#7878,.F.);
#10394=ORIENTED_EDGE('',*,*,#7879,.F.);
#10395=ORIENTED_EDGE('',*,*,#7880,.F.);
#10396=ORIENTED_EDGE('',*,*,#7881,.F.);
#10397=ORIENTED_EDGE('',*,*,#7882,.F.);
#10398=ORIENTED_EDGE('',*,*,#7883,.F.);
#10399=ORIENTED_EDGE('',*,*,#7884,.F.);
#10400=ORIENTED_EDGE('',*,*,#7885,.F.);
#10401=ORIENTED_EDGE('',*,*,#7886,.F.);
#10402=ORIENTED_EDGE('',*,*,#7887,.F.);
#10403=ORIENTED_EDGE('',*,*,#7888,.F.);
#10404=ORIENTED_EDGE('',*,*,#7889,.F.);
#10405=ORIENTED_EDGE('',*,*,#7890,.F.);
#10406=ORIENTED_EDGE('',*,*,#7891,.F.);
#10407=ORIENTED_EDGE('',*,*,#7892,.F.);
#10408=ORIENTED_EDGE('',*,*,#7893,.F.);
#10409=ORIENTED_EDGE('',*,*,#7876,.F.);
#10410=ORIENTED_EDGE('',*,*,#7874,.F.);
#10411=ORIENTED_EDGE('',*,*,#7894,.T.);
#10412=ORIENTED_EDGE('',*,*,#7895,.T.);
#10413=ORIENTED_EDGE('',*,*,#7896,.T.);
#10414=ORIENTED_EDGE('',*,*,#7894,.F.);
#10415=ORIENTED_EDGE('',*,*,#7897,.T.);
#10416=ORIENTED_EDGE('',*,*,#7898,.T.);
#10417=ORIENTED_EDGE('',*,*,#7891,.T.);
#10418=ORIENTED_EDGE('',*,*,#7898,.F.);
#10419=ORIENTED_EDGE('',*,*,#7897,.F.);
#10420=ORIENTED_EDGE('',*,*,#7899,.T.);
#10421=ORIENTED_EDGE('',*,*,#7900,.T.);
#10422=ORIENTED_EDGE('',*,*,#7901,.T.);
#10423=ORIENTED_EDGE('',*,*,#7899,.F.);
#10424=ORIENTED_EDGE('',*,*,#7902,.T.);
#10425=ORIENTED_EDGE('',*,*,#7903,.T.);
#10426=ORIENTED_EDGE('',*,*,#7893,.T.);
#10427=ORIENTED_EDGE('',*,*,#7903,.F.);
#10428=ORIENTED_EDGE('',*,*,#7902,.F.);
#10429=ORIENTED_EDGE('',*,*,#7904,.T.);
#10430=ORIENTED_EDGE('',*,*,#7905,.T.);
#10431=ORIENTED_EDGE('',*,*,#7906,.T.);
#10432=ORIENTED_EDGE('',*,*,#7904,.F.);
#10433=ORIENTED_EDGE('',*,*,#7907,.T.);
#10434=ORIENTED_EDGE('',*,*,#7908,.T.);
#10435=ORIENTED_EDGE('',*,*,#7892,.T.);
#10436=ORIENTED_EDGE('',*,*,#7908,.F.);
#10437=ORIENTED_EDGE('',*,*,#7907,.F.);
#10438=ORIENTED_EDGE('',*,*,#7909,.T.);
#10439=ORIENTED_EDGE('',*,*,#7910,.T.);
#10440=ORIENTED_EDGE('',*,*,#7911,.T.);
#10441=ORIENTED_EDGE('',*,*,#7909,.F.);
#10442=ORIENTED_EDGE('',*,*,#7912,.T.);
#10443=ORIENTED_EDGE('',*,*,#7895,.F.);
#10444=ORIENTED_EDGE('',*,*,#7896,.F.);
#10445=ORIENTED_EDGE('',*,*,#7912,.F.);
#10446=ORIENTED_EDGE('',*,*,#7913,.T.);
#10447=ORIENTED_EDGE('',*,*,#7910,.F.);
#10448=ORIENTED_EDGE('',*,*,#7911,.F.);
#10449=ORIENTED_EDGE('',*,*,#7913,.F.);
#10450=ORIENTED_EDGE('',*,*,#7914,.T.);
#10451=ORIENTED_EDGE('',*,*,#7905,.F.);
#10452=ORIENTED_EDGE('',*,*,#7906,.F.);
#10453=ORIENTED_EDGE('',*,*,#7914,.F.);
#10454=ORIENTED_EDGE('',*,*,#7915,.T.);
#10455=ORIENTED_EDGE('',*,*,#7900,.F.);
#10456=ORIENTED_EDGE('',*,*,#7901,.F.);
#10457=ORIENTED_EDGE('',*,*,#7915,.F.);
#10458=ORIENTED_EDGE('',*,*,#7916,.T.);
#10459=ORIENTED_EDGE('',*,*,#7917,.T.);
#10460=ORIENTED_EDGE('',*,*,#7918,.T.);
#10461=ORIENTED_EDGE('',*,*,#7917,.F.);
#10462=ORIENTED_EDGE('',*,*,#7919,.F.);
#10463=ORIENTED_EDGE('',*,*,#7920,.F.);
#10464=ORIENTED_EDGE('',*,*,#7921,.F.);
#10465=ORIENTED_EDGE('',*,*,#7922,.F.);
#10466=ORIENTED_EDGE('',*,*,#7923,.F.);
#10467=ORIENTED_EDGE('',*,*,#7924,.F.);
#10468=ORIENTED_EDGE('',*,*,#7925,.F.);
#10469=ORIENTED_EDGE('',*,*,#7926,.F.);
#10470=ORIENTED_EDGE('',*,*,#7927,.F.);
#10471=ORIENTED_EDGE('',*,*,#7928,.F.);
#10472=ORIENTED_EDGE('',*,*,#7929,.F.);
#10473=ORIENTED_EDGE('',*,*,#7930,.F.);
#10474=ORIENTED_EDGE('',*,*,#7931,.F.);
#10475=ORIENTED_EDGE('',*,*,#7932,.F.);
#10476=ORIENTED_EDGE('',*,*,#7933,.F.);
#10477=ORIENTED_EDGE('',*,*,#7934,.F.);
#10478=ORIENTED_EDGE('',*,*,#7935,.F.);
#10479=ORIENTED_EDGE('',*,*,#7918,.F.);
#10480=ORIENTED_EDGE('',*,*,#7916,.F.);
#10481=ORIENTED_EDGE('',*,*,#7936,.T.);
#10482=ORIENTED_EDGE('',*,*,#7937,.T.);
#10483=ORIENTED_EDGE('',*,*,#7936,.F.);
#10484=ORIENTED_EDGE('',*,*,#7938,.T.);
#10485=ORIENTED_EDGE('',*,*,#7939,.T.);
#10486=ORIENTED_EDGE('',*,*,#7923,.T.);
#10487=ORIENTED_EDGE('',*,*,#7939,.F.);
#10488=ORIENTED_EDGE('',*,*,#7938,.F.);
#10489=ORIENTED_EDGE('',*,*,#7940,.T.);
#10490=ORIENTED_EDGE('',*,*,#7941,.T.);
#10491=ORIENTED_EDGE('',*,*,#7940,.F.);
#10492=ORIENTED_EDGE('',*,*,#7942,.T.);
#10493=ORIENTED_EDGE('',*,*,#7943,.T.);
#10494=ORIENTED_EDGE('',*,*,#7935,.T.);
#10495=ORIENTED_EDGE('',*,*,#7943,.F.);
#10496=ORIENTED_EDGE('',*,*,#7942,.F.);
#10497=ORIENTED_EDGE('',*,*,#7944,.T.);
#10498=ORIENTED_EDGE('',*,*,#7945,.T.);
#10499=ORIENTED_EDGE('',*,*,#7944,.F.);
#10500=ORIENTED_EDGE('',*,*,#7946,.T.);
#10501=ORIENTED_EDGE('',*,*,#7947,.T.);
#10502=ORIENTED_EDGE('',*,*,#7924,.T.);
#10503=ORIENTED_EDGE('',*,*,#7947,.F.);
#10504=ORIENTED_EDGE('',*,*,#7946,.F.);
#10505=ORIENTED_EDGE('',*,*,#7948,.T.);
#10506=ORIENTED_EDGE('',*,*,#7949,.T.);
#10507=ORIENTED_EDGE('',*,*,#7948,.F.);
#10508=ORIENTED_EDGE('',*,*,#7950,.T.);
#10509=ORIENTED_EDGE('',*,*,#7951,.T.);
#10510=ORIENTED_EDGE('',*,*,#7934,.T.);
#10511=ORIENTED_EDGE('',*,*,#7951,.F.);
#10512=ORIENTED_EDGE('',*,*,#7950,.F.);
#10513=ORIENTED_EDGE('',*,*,#7952,.T.);
#10514=ORIENTED_EDGE('',*,*,#7953,.T.);
#10515=ORIENTED_EDGE('',*,*,#7952,.F.);
#10516=ORIENTED_EDGE('',*,*,#7954,.T.);
#10517=ORIENTED_EDGE('',*,*,#7955,.T.);
#10518=ORIENTED_EDGE('',*,*,#7925,.T.);
#10519=ORIENTED_EDGE('',*,*,#7955,.F.);
#10520=ORIENTED_EDGE('',*,*,#7954,.F.);
#10521=ORIENTED_EDGE('',*,*,#7956,.T.);
#10522=ORIENTED_EDGE('',*,*,#7957,.T.);
#10523=ORIENTED_EDGE('',*,*,#7956,.F.);
#10524=ORIENTED_EDGE('',*,*,#7958,.T.);
#10525=ORIENTED_EDGE('',*,*,#7937,.F.);
#10526=ORIENTED_EDGE('',*,*,#7958,.F.);
#10527=ORIENTED_EDGE('',*,*,#7959,.T.);
#10528=ORIENTED_EDGE('',*,*,#7957,.F.);
#10529=ORIENTED_EDGE('',*,*,#7959,.F.);
#10530=ORIENTED_EDGE('',*,*,#7960,.T.);
#10531=ORIENTED_EDGE('',*,*,#7941,.F.);
#10532=ORIENTED_EDGE('',*,*,#7960,.F.);
#10533=ORIENTED_EDGE('',*,*,#7961,.T.);
#10534=ORIENTED_EDGE('',*,*,#7945,.F.);
#10535=ORIENTED_EDGE('',*,*,#7961,.F.);
#10536=ORIENTED_EDGE('',*,*,#7962,.T.);
#10537=ORIENTED_EDGE('',*,*,#7949,.F.);
#10538=ORIENTED_EDGE('',*,*,#7962,.F.);
#10539=ORIENTED_EDGE('',*,*,#7963,.T.);
#10540=ORIENTED_EDGE('',*,*,#7953,.F.);
#10541=ORIENTED_EDGE('',*,*,#7963,.F.);
#10542=ORIENTED_EDGE('',*,*,#7964,.T.);
#10543=ORIENTED_EDGE('',*,*,#7965,.T.);
#10544=ORIENTED_EDGE('',*,*,#7926,.T.);
#10545=ORIENTED_EDGE('',*,*,#7965,.F.);
#10546=ORIENTED_EDGE('',*,*,#7964,.F.);
#10547=ORIENTED_EDGE('',*,*,#7966,.T.);
#10548=ORIENTED_EDGE('',*,*,#7967,.T.);
#10549=ORIENTED_EDGE('',*,*,#7966,.F.);
#10550=ORIENTED_EDGE('',*,*,#7968,.T.);
#10551=ORIENTED_EDGE('',*,*,#7969,.T.);
#10552=ORIENTED_EDGE('',*,*,#7933,.T.);
#10553=ORIENTED_EDGE('',*,*,#7969,.F.);
#10554=ORIENTED_EDGE('',*,*,#7968,.F.);
#10555=ORIENTED_EDGE('',*,*,#7970,.T.);
#10556=ORIENTED_EDGE('',*,*,#7971,.T.);
#10557=ORIENTED_EDGE('',*,*,#7970,.F.);
#10558=ORIENTED_EDGE('',*,*,#7972,.T.);
#10559=ORIENTED_EDGE('',*,*,#7973,.T.);
#10560=ORIENTED_EDGE('',*,*,#7927,.T.);
#10561=ORIENTED_EDGE('',*,*,#7973,.F.);
#10562=ORIENTED_EDGE('',*,*,#7972,.F.);
#10563=ORIENTED_EDGE('',*,*,#7974,.T.);
#10564=ORIENTED_EDGE('',*,*,#7975,.T.);
#10565=ORIENTED_EDGE('',*,*,#7974,.F.);
#10566=ORIENTED_EDGE('',*,*,#7976,.T.);
#10567=ORIENTED_EDGE('',*,*,#7977,.T.);
#10568=ORIENTED_EDGE('',*,*,#7932,.T.);
#10569=ORIENTED_EDGE('',*,*,#7977,.F.);
#10570=ORIENTED_EDGE('',*,*,#7976,.F.);
#10571=ORIENTED_EDGE('',*,*,#7978,.T.);
#10572=ORIENTED_EDGE('',*,*,#7979,.T.);
#10573=ORIENTED_EDGE('',*,*,#7978,.F.);
#10574=ORIENTED_EDGE('',*,*,#7980,.T.);
#10575=ORIENTED_EDGE('',*,*,#7981,.T.);
#10576=ORIENTED_EDGE('',*,*,#7928,.T.);
#10577=ORIENTED_EDGE('',*,*,#7981,.F.);
#10578=ORIENTED_EDGE('',*,*,#7980,.F.);
#10579=ORIENTED_EDGE('',*,*,#7982,.T.);
#10580=ORIENTED_EDGE('',*,*,#7983,.T.);
#10581=ORIENTED_EDGE('',*,*,#7982,.F.);
#10582=ORIENTED_EDGE('',*,*,#7984,.T.);
#10583=ORIENTED_EDGE('',*,*,#7985,.T.);
#10584=ORIENTED_EDGE('',*,*,#7931,.T.);
#10585=ORIENTED_EDGE('',*,*,#7985,.F.);
#10586=ORIENTED_EDGE('',*,*,#7984,.F.);
#10587=ORIENTED_EDGE('',*,*,#7986,.T.);
#10588=ORIENTED_EDGE('',*,*,#7987,.T.);
#10589=ORIENTED_EDGE('',*,*,#7986,.F.);
#10590=ORIENTED_EDGE('',*,*,#7988,.T.);
#10591=ORIENTED_EDGE('',*,*,#7989,.T.);
#10592=ORIENTED_EDGE('',*,*,#7929,.T.);
#10593=ORIENTED_EDGE('',*,*,#7989,.F.);
#10594=ORIENTED_EDGE('',*,*,#7988,.F.);
#10595=ORIENTED_EDGE('',*,*,#7990,.T.);
#10596=ORIENTED_EDGE('',*,*,#7991,.T.);
#10597=ORIENTED_EDGE('',*,*,#7990,.F.);
#10598=ORIENTED_EDGE('',*,*,#7992,.T.);
#10599=ORIENTED_EDGE('',*,*,#7993,.T.);
#10600=ORIENTED_EDGE('',*,*,#7930,.T.);
#10601=ORIENTED_EDGE('',*,*,#7993,.F.);
#10602=ORIENTED_EDGE('',*,*,#7992,.F.);
#10603=ORIENTED_EDGE('',*,*,#7994,.T.);
#10604=ORIENTED_EDGE('',*,*,#7995,.T.);
#10605=ORIENTED_EDGE('',*,*,#7994,.F.);
#10606=ORIENTED_EDGE('',*,*,#7995,.F.);
#10607=ORIENTED_EDGE('',*,*,#7996,.F.);
#10608=ORIENTED_EDGE('',*,*,#7991,.F.);
#10609=ORIENTED_EDGE('',*,*,#7997,.F.);
#10610=ORIENTED_EDGE('',*,*,#7987,.F.);
#10611=ORIENTED_EDGE('',*,*,#7998,.F.);
#10612=ORIENTED_EDGE('',*,*,#7983,.F.);
#10613=ORIENTED_EDGE('',*,*,#7999,.F.);
#10614=ORIENTED_EDGE('',*,*,#7979,.F.);
#10615=ORIENTED_EDGE('',*,*,#8000,.F.);
#10616=ORIENTED_EDGE('',*,*,#7975,.F.);
#10617=ORIENTED_EDGE('',*,*,#8001,.F.);
#10618=ORIENTED_EDGE('',*,*,#7971,.F.);
#10619=ORIENTED_EDGE('',*,*,#8002,.F.);
#10620=ORIENTED_EDGE('',*,*,#7967,.F.);
#10621=ORIENTED_EDGE('',*,*,#8003,.F.);
#10622=ORIENTED_EDGE('',*,*,#7996,.T.);
#10623=ORIENTED_EDGE('',*,*,#8004,.T.);
#10624=ORIENTED_EDGE('',*,*,#8005,.F.);
#10625=ORIENTED_EDGE('',*,*,#8004,.F.);
#10626=ORIENTED_EDGE('',*,*,#7997,.T.);
#10627=ORIENTED_EDGE('',*,*,#8006,.T.);
#10628=ORIENTED_EDGE('',*,*,#8007,.F.);
#10629=ORIENTED_EDGE('',*,*,#8006,.F.);
#10630=ORIENTED_EDGE('',*,*,#7998,.T.);
#10631=ORIENTED_EDGE('',*,*,#8008,.T.);
#10632=ORIENTED_EDGE('',*,*,#8009,.F.);
#10633=ORIENTED_EDGE('',*,*,#8008,.F.);
#10634=ORIENTED_EDGE('',*,*,#7999,.T.);
#10635=ORIENTED_EDGE('',*,*,#8010,.T.);
#10636=ORIENTED_EDGE('',*,*,#8011,.F.);
#10637=ORIENTED_EDGE('',*,*,#8010,.F.);
#10638=ORIENTED_EDGE('',*,*,#8000,.T.);
#10639=ORIENTED_EDGE('',*,*,#8012,.T.);
#10640=ORIENTED_EDGE('',*,*,#8013,.F.);
#10641=ORIENTED_EDGE('',*,*,#8012,.F.);
#10642=ORIENTED_EDGE('',*,*,#8001,.T.);
#10643=ORIENTED_EDGE('',*,*,#8014,.T.);
#10644=ORIENTED_EDGE('',*,*,#8015,.F.);
#10645=ORIENTED_EDGE('',*,*,#8014,.F.);
#10646=ORIENTED_EDGE('',*,*,#8002,.T.);
#10647=ORIENTED_EDGE('',*,*,#8016,.T.);
#10648=ORIENTED_EDGE('',*,*,#8017,.F.);
#10649=ORIENTED_EDGE('',*,*,#8016,.F.);
#10650=ORIENTED_EDGE('',*,*,#8003,.T.);
#10651=ORIENTED_EDGE('',*,*,#8018,.T.);
#10652=ORIENTED_EDGE('',*,*,#8019,.F.);
#10653=ORIENTED_EDGE('',*,*,#8018,.F.);
#10654=ORIENTED_EDGE('',*,*,#8020,.T.);
#10655=ORIENTED_EDGE('',*,*,#7835,.T.);
#10656=ORIENTED_EDGE('',*,*,#8021,.T.);
#10657=ORIENTED_EDGE('',*,*,#8022,.T.);
#10658=ORIENTED_EDGE('',*,*,#7761,.T.);
#10659=ORIENTED_EDGE('',*,*,#8021,.F.);
#10660=ORIENTED_EDGE('',*,*,#7848,.T.);
#10661=ORIENTED_EDGE('',*,*,#8023,.T.);
#10662=ORIENTED_EDGE('',*,*,#8024,.T.);
#10663=ORIENTED_EDGE('',*,*,#7919,.T.);
#10664=ORIENTED_EDGE('',*,*,#8025,.T.);
#10665=ORIENTED_EDGE('',*,*,#8020,.F.);
#10666=ORIENTED_EDGE('',*,*,#7764,.T.);
#10667=ORIENTED_EDGE('',*,*,#8026,.F.);
#10668=ORIENTED_EDGE('',*,*,#8027,.T.);
#10669=ORIENTED_EDGE('',*,*,#8024,.F.);
#10670=ORIENTED_EDGE('',*,*,#8028,.F.);
#10671=ORIENTED_EDGE('',*,*,#7816,.T.);
#10672=ORIENTED_EDGE('',*,*,#8029,.F.);
#10673=ORIENTED_EDGE('',*,*,#8030,.F.);
#10674=ORIENTED_EDGE('',*,*,#7920,.T.);
#10675=ORIENTED_EDGE('',*,*,#8023,.F.);
#10676=ORIENTED_EDGE('',*,*,#7847,.T.);
#10677=ORIENTED_EDGE('',*,*,#8031,.T.);
#10678=ORIENTED_EDGE('',*,*,#7813,.T.);
#10679=ORIENTED_EDGE('',*,*,#8028,.T.);
#10680=ORIENTED_EDGE('',*,*,#8029,.T.);
#10681=ORIENTED_EDGE('',*,*,#7815,.T.);
#10682=ORIENTED_EDGE('',*,*,#8032,.T.);
#10683=ORIENTED_EDGE('',*,*,#7877,.T.);
#10684=ORIENTED_EDGE('',*,*,#8033,.T.);
#10685=ORIENTED_EDGE('',*,*,#8033,.F.);
#10686=ORIENTED_EDGE('',*,*,#7890,.T.);
#10687=ORIENTED_EDGE('',*,*,#8034,.T.);
#10688=ORIENTED_EDGE('',*,*,#8035,.T.);
#10689=ORIENTED_EDGE('',*,*,#7921,.T.);
#10690=ORIENTED_EDGE('',*,*,#8030,.T.);
#10691=ORIENTED_EDGE('',*,*,#8022,.F.);
#10692=ORIENTED_EDGE('',*,*,#8025,.F.);
#10693=ORIENTED_EDGE('',*,*,#7922,.T.);
#10694=ORIENTED_EDGE('',*,*,#8035,.F.);
#10695=ORIENTED_EDGE('',*,*,#8036,.F.);
#10696=ORIENTED_EDGE('',*,*,#7762,.T.);
#10697=ORIENTED_EDGE('',*,*,#8034,.F.);
#10698=ORIENTED_EDGE('',*,*,#7889,.T.);
#10699=ORIENTED_EDGE('',*,*,#8026,.T.);
#10700=ORIENTED_EDGE('',*,*,#7763,.T.);
#10701=ORIENTED_EDGE('',*,*,#8036,.T.);
#10702=ORIENTED_EDGE('',*,*,#7845,.T.);
#10703=ORIENTED_EDGE('',*,*,#8037,.T.);
#10704=ORIENTED_EDGE('',*,*,#7879,.T.);
#10705=ORIENTED_EDGE('',*,*,#8038,.T.);
#10706=ORIENTED_EDGE('',*,*,#8038,.F.);
#10707=ORIENTED_EDGE('',*,*,#7878,.T.);
#10708=ORIENTED_EDGE('',*,*,#8039,.F.);
#10709=ORIENTED_EDGE('',*,*,#7846,.F.);
#10710=ORIENTED_EDGE('',*,*,#8005,.T.);
#10711=ORIENTED_EDGE('',*,*,#8007,.T.);
#10712=ORIENTED_EDGE('',*,*,#8013,.T.);
#10713=ORIENTED_EDGE('',*,*,#8015,.T.);
#10714=ORIENTED_EDGE('',*,*,#7837,.T.);
#10715=ORIENTED_EDGE('',*,*,#8040,.T.);
#10716=ORIENTED_EDGE('',*,*,#7887,.T.);
#10717=ORIENTED_EDGE('',*,*,#8041,.T.);
#10718=ORIENTED_EDGE('',*,*,#8041,.F.);
#10719=ORIENTED_EDGE('',*,*,#7886,.T.);
#10720=ORIENTED_EDGE('',*,*,#8042,.T.);
#10721=ORIENTED_EDGE('',*,*,#7838,.F.);
#10722=ORIENTED_EDGE('',*,*,#7779,.T.);
#10723=ORIENTED_EDGE('',*,*,#7777,.T.);
#10724=ORIENTED_EDGE('',*,*,#7775,.T.);
#10725=ORIENTED_EDGE('',*,*,#7738,.T.);
#10726=ORIENTED_EDGE('',*,*,#7749,.T.);
#10727=ORIENTED_EDGE('',*,*,#7760,.T.);
#10728=ORIENTED_EDGE('',*,*,#8031,.F.);
#10729=ORIENTED_EDGE('',*,*,#8039,.T.);
#10730=ORIENTED_EDGE('',*,*,#8032,.F.);
#10731=ORIENTED_EDGE('',*,*,#7814,.T.);
#10732=ORIENTED_EDGE('',*,*,#8040,.F.);
#10733=ORIENTED_EDGE('',*,*,#7836,.F.);
#10734=ORIENTED_EDGE('',*,*,#8027,.F.);
#10735=ORIENTED_EDGE('',*,*,#7888,.T.);
#10736=ORIENTED_EDGE('',*,*,#8009,.T.);
#10737=ORIENTED_EDGE('',*,*,#8011,.T.);
#10738=ORIENTED_EDGE('',*,*,#8017,.T.);
#10739=ORIENTED_EDGE('',*,*,#8019,.T.);
#10740=ORIENTED_EDGE('',*,*,#8037,.F.);
#10741=ORIENTED_EDGE('',*,*,#7844,.F.);
#10742=ORIENTED_EDGE('',*,*,#8043,.F.);
#10743=ORIENTED_EDGE('',*,*,#7880,.T.);
#10744=ORIENTED_EDGE('',*,*,#7831,.T.);
#10745=ORIENTED_EDGE('',*,*,#7829,.T.);
#10746=ORIENTED_EDGE('',*,*,#7827,.T.);
#10747=ORIENTED_EDGE('',*,*,#7790,.T.);
#10748=ORIENTED_EDGE('',*,*,#7801,.T.);
#10749=ORIENTED_EDGE('',*,*,#7812,.T.);
#10750=ORIENTED_EDGE('',*,*,#7881,.T.);
#10751=ORIENTED_EDGE('',*,*,#8043,.T.);
#10752=ORIENTED_EDGE('',*,*,#7843,.F.);
#10753=ORIENTED_EDGE('',*,*,#8044,.F.);
#10754=ORIENTED_EDGE('',*,*,#7882,.T.);
#10755=ORIENTED_EDGE('',*,*,#8044,.T.);
#10756=ORIENTED_EDGE('',*,*,#7842,.F.);
#10757=ORIENTED_EDGE('',*,*,#8045,.F.);
#10758=ORIENTED_EDGE('',*,*,#7883,.T.);
#10759=ORIENTED_EDGE('',*,*,#8045,.T.);
#10760=ORIENTED_EDGE('',*,*,#7841,.F.);
#10761=ORIENTED_EDGE('',*,*,#8046,.F.);
#10762=ORIENTED_EDGE('',*,*,#7884,.T.);
#10763=ORIENTED_EDGE('',*,*,#8046,.T.);
#10764=ORIENTED_EDGE('',*,*,#7840,.F.);
#10765=ORIENTED_EDGE('',*,*,#8047,.F.);
#10766=ORIENTED_EDGE('',*,*,#7885,.T.);
#10767=ORIENTED_EDGE('',*,*,#8047,.T.);
#10768=ORIENTED_EDGE('',*,*,#7839,.F.);
#10769=ORIENTED_EDGE('',*,*,#8042,.F.);
#14262=CONICAL_SURFACE('',#15328,2.7,0.785398163397448);
#14263=CONICAL_SURFACE('',#15332,5.15000000000001,0.785398163397478);
#14264=CONICAL_SURFACE('',#15338,2.7,0.785398163397448);
#14265=CONICAL_SURFACE('',#15342,5.15,0.785398163397448);
#14266=CONICAL_SURFACE('',#15348,2.7,0.785398163397463);
#14267=CONICAL_SURFACE('',#15352,5.15,0.785398163397463);
#14268=CONICAL_SURFACE('',#15377,2.7,0.785398163397438);
#14269=CONICAL_SURFACE('',#15381,5.15000000000001,0.785398163397467);
#14270=CONICAL_SURFACE('',#15387,2.7,0.785398163397438);
#14271=CONICAL_SURFACE('',#15391,5.15,0.785398163397438);
#14272=CONICAL_SURFACE('',#15397,2.7,0.785398163397452);
#14273=CONICAL_SURFACE('',#15401,5.15,0.785398163397452);
#14274=CONICAL_SURFACE('',#15426,2.2,0.785398163397419);
#14275=CONICAL_SURFACE('',#15436,2.2,0.78539816339743);
#14276=CONICAL_SURFACE('',#15441,2.2,0.785398163397434);
#14277=CONICAL_SURFACE('',#15446,2.2,0.785398163397429);
#14278=CONICAL_SURFACE('',#15451,1.025,1.02974425867666);
#14279=CONICAL_SURFACE('',#15452,1.025,1.02974425867666);
#14280=CONICAL_SURFACE('',#15453,1.025,1.02974425867666);
#14281=CONICAL_SURFACE('',#15454,1.025,1.02974425867666);
#14282=CONICAL_SURFACE('',#15455,2.2,0.785398163397438);
#14283=CONICAL_SURFACE('',#15465,2.2,0.785398163397449);
#14284=CONICAL_SURFACE('',#15470,2.2,0.785398163397452);
#14285=CONICAL_SURFACE('',#15475,2.2,0.785398163397448);
#14286=CONICAL_SURFACE('',#15480,2.05,1.02974425867665);
#14287=CONICAL_SURFACE('',#15481,2.05,1.02974425867665);
#14288=CONICAL_SURFACE('',#15482,2.05,1.02974425867665);
#14289=CONICAL_SURFACE('',#15483,2.05,1.02974425867665);
#14290=CONICAL_SURFACE('',#15484,3.24999999999999,0.785398163397437);
#14291=CONICAL_SURFACE('',#15503,3.24999999999999,0.785398163397437);
#14292=CONICAL_SURFACE('',#15507,3.24999999999999,0.785398163397437);
#14293=CONICAL_SURFACE('',#15511,3.25,0.785398163397448);
#14294=CONICAL_SURFACE('',#15515,3.25,0.785398163397448);
#14295=CONICAL_SURFACE('',#15519,3.24999999999999,0.785398163397437);
#14296=CONICAL_SURFACE('',#15523,3.05000000000001,1.02974425867666);
#14297=CONICAL_SURFACE('',#15524,3.05000000000001,1.02974425867666);
#14298=CONICAL_SURFACE('',#15525,3.05,1.02974425867665);
#14299=CONICAL_SURFACE('',#15526,3.05,1.02974425867665);
#14300=CONICAL_SURFACE('',#15527,3.05,1.02974425867665);
#14301=CONICAL_SURFACE('',#15528,3.05,1.02974425867665);
#14302=CONICAL_SURFACE('',#15529,5.65000000000001,0.785398163397463);
#14303=CONICAL_SURFACE('',#15533,5.65,0.785398163397434);
#14304=CONICAL_SURFACE('',#15537,5.65,0.785398163397441);
#14305=CONICAL_SURFACE('',#15541,5.65,0.785398163397434);
#14306=CONICAL_SURFACE('',#15545,5.65,0.785398163397441);
#14307=CONICAL_SURFACE('',#15549,5.65,0.785398163397434);
#14308=CONICAL_SURFACE('',#15553,5.65,0.785398163397434);
#14309=CONICAL_SURFACE('',#15557,5.65000000000001,0.785398163397463);
#14413=ADVANCED_FACE('',(#1678),#14262,.F.);
#14414=ADVANCED_FACE('',(#1679),#14263,.F.);
#14415=ADVANCED_FACE('',(#1680),#867,.F.);
#14416=ADVANCED_FACE('',(#1681),#14264,.F.);
#14417=ADVANCED_FACE('',(#1682),#14265,.F.);
#14418=ADVANCED_FACE('',(#1683),#868,.F.);
#14419=ADVANCED_FACE('',(#1684),#14266,.F.);
#14420=ADVANCED_FACE('',(#1685),#14267,.F.);
#14421=ADVANCED_FACE('',(#1686),#869,.F.);
#14422=ADVANCED_FACE('',(#1687,#1107,#1108,#1109),#1243,.T.);
#14423=ADVANCED_FACE('',(#1688),#870,.F.);
#14424=ADVANCED_FACE('',(#1689),#871,.F.);
#14425=ADVANCED_FACE('',(#1690),#872,.F.);
#14426=ADVANCED_FACE('',(#1691,#1110),#1244,.T.);
#14427=ADVANCED_FACE('',(#1692,#1111),#1245,.T.);
#14428=ADVANCED_FACE('',(#1693,#1112),#1246,.T.);
#14429=ADVANCED_FACE('',(#1694),#873,.F.);
#14430=ADVANCED_FACE('',(#1695),#874,.F.);
#14431=ADVANCED_FACE('',(#1696),#875,.F.);
#14432=ADVANCED_FACE('',(#1697),#14268,.F.);
#14433=ADVANCED_FACE('',(#1698),#14269,.F.);
#14434=ADVANCED_FACE('',(#1699),#876,.F.);
#14435=ADVANCED_FACE('',(#1700),#14270,.F.);
#14436=ADVANCED_FACE('',(#1701),#14271,.F.);
#14437=ADVANCED_FACE('',(#1702),#877,.F.);
#14438=ADVANCED_FACE('',(#1703),#14272,.F.);
#14439=ADVANCED_FACE('',(#1704),#14273,.F.);
#14440=ADVANCED_FACE('',(#1705),#878,.F.);
#14441=ADVANCED_FACE('',(#1706,#1113,#1114,#1115),#1247,.T.);
#14442=ADVANCED_FACE('',(#1707),#879,.F.);
#14443=ADVANCED_FACE('',(#1708),#880,.F.);
#14444=ADVANCED_FACE('',(#1709),#881,.F.);
#14445=ADVANCED_FACE('',(#1710,#1116),#1248,.F.);
#14446=ADVANCED_FACE('',(#1711,#1117),#1249,.F.);
#14447=ADVANCED_FACE('',(#1712,#1118),#1250,.F.);
#14448=ADVANCED_FACE('',(#1713),#882,.F.);
#14449=ADVANCED_FACE('',(#1714),#883,.F.);
#14450=ADVANCED_FACE('',(#1715),#884,.F.);
#14451=ADVANCED_FACE('',(#1716),#14274,.F.);
#14452=ADVANCED_FACE('',(#1717,#1119,#1120,#1121,#1122),#1251,.T.);
#14453=ADVANCED_FACE('',(#1718),#885,.F.);
#14454=ADVANCED_FACE('',(#1719),#14275,.F.);
#14455=ADVANCED_FACE('',(#1720),#886,.F.);
#14456=ADVANCED_FACE('',(#1721),#14276,.F.);
#14457=ADVANCED_FACE('',(#1722),#887,.F.);
#14458=ADVANCED_FACE('',(#1723),#14277,.F.);
#14459=ADVANCED_FACE('',(#1724),#888,.F.);
#14460=ADVANCED_FACE('',(#1725),#14278,.F.);
#14461=ADVANCED_FACE('',(#1726),#14279,.F.);
#14462=ADVANCED_FACE('',(#1727),#14280,.F.);
#14463=ADVANCED_FACE('',(#1728),#14281,.F.);
#14464=ADVANCED_FACE('',(#1729),#14282,.F.);
#14465=ADVANCED_FACE('',(#1730,#1123,#1124,#1125,#1126),#1252,.F.);
#14466=ADVANCED_FACE('',(#1731),#889,.F.);
#14467=ADVANCED_FACE('',(#1732),#14283,.F.);
#14468=ADVANCED_FACE('',(#1733),#890,.F.);
#14469=ADVANCED_FACE('',(#1734),#14284,.F.);
#14470=ADVANCED_FACE('',(#1735),#891,.F.);
#14471=ADVANCED_FACE('',(#1736),#14285,.F.);
#14472=ADVANCED_FACE('',(#1737),#892,.F.);
#14473=ADVANCED_FACE('',(#1738),#14286,.F.);
#14474=ADVANCED_FACE('',(#1739),#14287,.F.);
#14475=ADVANCED_FACE('',(#1740),#14288,.F.);
#14476=ADVANCED_FACE('',(#1741),#14289,.F.);
#14477=ADVANCED_FACE('',(#1742),#14290,.F.);
#14478=ADVANCED_FACE('',(#1743,#1127,#1128,#1129,#1130,#1131,#1132,#1133,
#1134,#1135,#1136,#1137,#1138,#1139,#1140),#1253,.T.);
#14479=ADVANCED_FACE('',(#1744),#893,.F.);
#14480=ADVANCED_FACE('',(#1745),#14291,.F.);
#14481=ADVANCED_FACE('',(#1746),#894,.F.);
#14482=ADVANCED_FACE('',(#1747),#14292,.F.);
#14483=ADVANCED_FACE('',(#1748),#895,.F.);
#14484=ADVANCED_FACE('',(#1749),#14293,.F.);
#14485=ADVANCED_FACE('',(#1750),#896,.F.);
#14486=ADVANCED_FACE('',(#1751),#14294,.F.);
#14487=ADVANCED_FACE('',(#1752),#897,.F.);
#14488=ADVANCED_FACE('',(#1753),#14295,.F.);
#14489=ADVANCED_FACE('',(#1754),#898,.F.);
#14490=ADVANCED_FACE('',(#1755),#14296,.F.);
#14491=ADVANCED_FACE('',(#1756),#14297,.F.);
#14492=ADVANCED_FACE('',(#1757),#14298,.F.);
#14493=ADVANCED_FACE('',(#1758),#14299,.F.);
#14494=ADVANCED_FACE('',(#1759),#14300,.F.);
#14495=ADVANCED_FACE('',(#1760),#14301,.F.);
#14496=ADVANCED_FACE('',(#1761),#14302,.F.);
#14497=ADVANCED_FACE('',(#1762),#899,.F.);
#14498=ADVANCED_FACE('',(#1763),#14303,.F.);
#14499=ADVANCED_FACE('',(#1764),#900,.F.);
#14500=ADVANCED_FACE('',(#1765),#14304,.F.);
#14501=ADVANCED_FACE('',(#1766),#901,.F.);
#14502=ADVANCED_FACE('',(#1767),#14305,.F.);
#14503=ADVANCED_FACE('',(#1768),#902,.F.);
#14504=ADVANCED_FACE('',(#1769),#14306,.F.);
#14505=ADVANCED_FACE('',(#1770),#903,.F.);
#14506=ADVANCED_FACE('',(#1771),#14307,.F.);
#14507=ADVANCED_FACE('',(#1772),#904,.F.);
#14508=ADVANCED_FACE('',(#1773),#14308,.F.);
#14509=ADVANCED_FACE('',(#1774),#905,.F.);
#14510=ADVANCED_FACE('',(#1775),#14309,.F.);
#14511=ADVANCED_FACE('',(#1776),#906,.F.);
#14512=ADVANCED_FACE('',(#1777,#1141),#1254,.T.);
#14513=ADVANCED_FACE('',(#1778,#1142),#1255,.T.);
#14514=ADVANCED_FACE('',(#1779,#1143),#1256,.T.);
#14515=ADVANCED_FACE('',(#1780,#1144),#1257,.T.);
#14516=ADVANCED_FACE('',(#1781,#1145),#1258,.T.);
#14517=ADVANCED_FACE('',(#1782,#1146),#1259,.T.);
#14518=ADVANCED_FACE('',(#1783,#1147),#1260,.T.);
#14519=ADVANCED_FACE('',(#1784,#1148),#1261,.T.);
#14520=ADVANCED_FACE('',(#1785),#907,.F.);
#14521=ADVANCED_FACE('',(#1786),#908,.F.);
#14522=ADVANCED_FACE('',(#1787),#909,.F.);
#14523=ADVANCED_FACE('',(#1788),#910,.F.);
#14524=ADVANCED_FACE('',(#1789),#911,.F.);
#14525=ADVANCED_FACE('',(#1790),#912,.F.);
#14526=ADVANCED_FACE('',(#1791),#913,.F.);
#14527=ADVANCED_FACE('',(#1792),#914,.F.);
#14528=ADVANCED_FACE('',(#1793),#1262,.T.);
#14529=ADVANCED_FACE('',(#1794),#1263,.T.);
#14530=ADVANCED_FACE('',(#1795),#1264,.T.);
#14531=ADVANCED_FACE('',(#1796),#1265,.T.);
#14532=ADVANCED_FACE('',(#1797),#1266,.T.);
#14533=ADVANCED_FACE('',(#1798),#1267,.T.);
#14534=ADVANCED_FACE('',(#1799),#1268,.T.);
#14535=ADVANCED_FACE('',(#1800),#1269,.T.);
#14536=ADVANCED_FACE('',(#1801),#1270,.T.);
#14537=ADVANCED_FACE('',(#1802),#1271,.T.);
#14538=ADVANCED_FACE('',(#1803,#1149,#1150,#1151,#1152),#1272,.T.);
#14539=ADVANCED_FACE('',(#1804),#1273,.T.);
#14540=ADVANCED_FACE('',(#1805,#1153,#1154,#1155,#1156,#1157,#1158),#1274,
 .T.);
#14541=ADVANCED_FACE('',(#1806),#1275,.T.);
#14542=ADVANCED_FACE('',(#1807,#1159,#1160,#1161,#1162),#1276,.T.);
#14543=ADVANCED_FACE('',(#1808,#1163,#1164,#1165,#1166,#1167,#1168),#1277,
 .T.);
#14544=ADVANCED_FACE('',(#1809),#1278,.T.);
#14545=ADVANCED_FACE('',(#1810),#1279,.T.);
#14546=ADVANCED_FACE('',(#1811),#1280,.T.);
#14547=ADVANCED_FACE('',(#1812),#1281,.T.);
#14548=ADVANCED_FACE('',(#1813),#1282,.T.);
#15085=CLOSED_SHELL('',(#14413,#14414,#14415,#14416,#14417,#14418,#14419,
#14420,#14421,#14422,#14423,#14424,#14425,#14426,#14427,#14428,#14429,#14430,
#14431,#14432,#14433,#14434,#14435,#14436,#14437,#14438,#14439,#14440,#14441,
#14442,#14443,#14444,#14445,#14446,#14447,#14448,#14449,#14450,#14451,#14452,
#14453,#14454,#14455,#14456,#14457,#14458,#14459,#14460,#14461,#14462,#14463,
#14464,#14465,#14466,#14467,#14468,#14469,#14470,#14471,#14472,#14473,#14474,
#14475,#14476,#14477,#14478,#14479,#14480,#14481,#14482,#14483,#14484,#14485,
#14486,#14487,#14488,#14489,#14490,#14491,#14492,#14493,#14494,#14495,#14496,
#14497,#14498,#14499,#14500,#14501,#14502,#14503,#14504,#14505,#14506,#14507,
#14508,#14509,#14510,#14511,#14512,#14513,#14514,#14515,#14516,#14517,#14518,
#14519,#14520,#14521,#14522,#14523,#14524,#14525,#14526,#14527,#14528,#14529,
#14530,#14531,#14532,#14533,#14534,#14535,#14536,#14537,#14538,#14539,#14540,
#14541,#14542,#14543,#14544,#14545,#14546,#14547,#14548));
#15327=AXIS2_PLACEMENT_3D('',#20922,#16990,#16991);
#15328=AXIS2_PLACEMENT_3D('',#20923,#16992,#16993);
#15329=AXIS2_PLACEMENT_3D('',#20925,#16994,#16995);
#15330=AXIS2_PLACEMENT_3D('',#20929,#16997,#16998);
#15331=AXIS2_PLACEMENT_3D('',#20937,#16999,#17000);
#15332=AXIS2_PLACEMENT_3D('',#20938,#17001,#17002);
#15333=AXIS2_PLACEMENT_3D('',#20940,#17003,#17004);
#15334=AXIS2_PLACEMENT_3D('',#20943,#17006,#17007);
#15335=AXIS2_PLACEMENT_3D('',#20944,#17008,#17009);
#15336=AXIS2_PLACEMENT_3D('',#20945,#17010,#17011);
#15337=AXIS2_PLACEMENT_3D('',#20948,#17013,#17014);
#15338=AXIS2_PLACEMENT_3D('',#20949,#17015,#17016);
#15339=AXIS2_PLACEMENT_3D('',#20951,#17017,#17018);
#15340=AXIS2_PLACEMENT_3D('',#20955,#17020,#17021);
#15341=AXIS2_PLACEMENT_3D('',#20963,#17022,#17023);
#15342=AXIS2_PLACEMENT_3D('',#20964,#17024,#17025);
#15343=AXIS2_PLACEMENT_3D('',#20966,#17026,#17027);
#15344=AXIS2_PLACEMENT_3D('',#20969,#17029,#17030);
#15345=AXIS2_PLACEMENT_3D('',#20970,#17031,#17032);
#15346=AXIS2_PLACEMENT_3D('',#20971,#17033,#17034);
#15347=AXIS2_PLACEMENT_3D('',#20974,#17036,#17037);
#15348=AXIS2_PLACEMENT_3D('',#20975,#17038,#17039);
#15349=AXIS2_PLACEMENT_3D('',#20977,#17040,#17041);
#15350=AXIS2_PLACEMENT_3D('',#20981,#17043,#17044);
#15351=AXIS2_PLACEMENT_3D('',#20989,#17045,#17046);
#15352=AXIS2_PLACEMENT_3D('',#20990,#17047,#17048);
#15353=AXIS2_PLACEMENT_3D('',#20992,#17049,#17050);
#15354=AXIS2_PLACEMENT_3D('',#20995,#17052,#17053);
#15355=AXIS2_PLACEMENT_3D('',#20996,#17054,#17055);
#15356=AXIS2_PLACEMENT_3D('',#20997,#17056,#17057);
#15357=AXIS2_PLACEMENT_3D('',#21000,#17059,#17060);
#15358=AXIS2_PLACEMENT_3D('',#21001,#17061,#17062);
#15359=AXIS2_PLACEMENT_3D('',#21010,#17067,#17068);
#15360=AXIS2_PLACEMENT_3D('',#21013,#17070,#17071);
#15361=AXIS2_PLACEMENT_3D('',#21014,#17072,#17073);
#15362=AXIS2_PLACEMENT_3D('',#21017,#17075,#17076);
#15363=AXIS2_PLACEMENT_3D('',#21018,#17077,#17078);
#15364=AXIS2_PLACEMENT_3D('',#21021,#17080,#17081);
#15365=AXIS2_PLACEMENT_3D('',#21022,#17082,#17083);
#15366=AXIS2_PLACEMENT_3D('',#21024,#17084,#17085);
#15367=AXIS2_PLACEMENT_3D('',#21025,#17086,#17087);
#15368=AXIS2_PLACEMENT_3D('',#21027,#17088,#17089);
#15369=AXIS2_PLACEMENT_3D('',#21028,#17090,#17091);
#15370=AXIS2_PLACEMENT_3D('',#21030,#17092,#17093);
#15371=AXIS2_PLACEMENT_3D('',#21031,#17094,#17095);
#15372=AXIS2_PLACEMENT_3D('',#21034,#17097,#17098);
#15373=AXIS2_PLACEMENT_3D('',#21035,#17099,#17100);
#15374=AXIS2_PLACEMENT_3D('',#21038,#17102,#17103);
#15375=AXIS2_PLACEMENT_3D('',#21039,#17104,#17105);
#15376=AXIS2_PLACEMENT_3D('',#21042,#17107,#17108);
#15377=AXIS2_PLACEMENT_3D('',#21043,#17109,#17110);
#15378=AXIS2_PLACEMENT_3D('',#21045,#17111,#17112);
#15379=AXIS2_PLACEMENT_3D('',#21049,#17114,#17115);
#15380=AXIS2_PLACEMENT_3D('',#21057,#17116,#17117);
#15381=AXIS2_PLACEMENT_3D('',#21058,#17118,#17119);
#15382=AXIS2_PLACEMENT_3D('',#21060,#17120,#17121);
#15383=AXIS2_PLACEMENT_3D('',#21063,#17123,#17124);
#15384=AXIS2_PLACEMENT_3D('',#21064,#17125,#17126);
#15385=AXIS2_PLACEMENT_3D('',#21065,#17127,#17128);
#15386=AXIS2_PLACEMENT_3D('',#21068,#17130,#17131);
#15387=AXIS2_PLACEMENT_3D('',#21069,#17132,#17133);
#15388=AXIS2_PLACEMENT_3D('',#21071,#17134,#17135);
#15389=AXIS2_PLACEMENT_3D('',#21075,#17137,#17138);
#15390=AXIS2_PLACEMENT_3D('',#21083,#17139,#17140);
#15391=AXIS2_PLACEMENT_3D('',#21084,#17141,#17142);
#15392=AXIS2_PLACEMENT_3D('',#21086,#17143,#17144);
#15393=AXIS2_PLACEMENT_3D('',#21089,#17146,#17147);
#15394=AXIS2_PLACEMENT_3D('',#21090,#17148,#17149);
#15395=AXIS2_PLACEMENT_3D('',#21091,#17150,#17151);
#15396=AXIS2_PLACEMENT_3D('',#21094,#17153,#17154);
#15397=AXIS2_PLACEMENT_3D('',#21095,#17155,#17156);
#15398=AXIS2_PLACEMENT_3D('',#21097,#17157,#17158);
#15399=AXIS2_PLACEMENT_3D('',#21101,#17160,#17161);
#15400=AXIS2_PLACEMENT_3D('',#21109,#17162,#17163);
#15401=AXIS2_PLACEMENT_3D('',#21110,#17164,#17165);
#15402=AXIS2_PLACEMENT_3D('',#21112,#17166,#17167);
#15403=AXIS2_PLACEMENT_3D('',#21115,#17169,#17170);
#15404=AXIS2_PLACEMENT_3D('',#21116,#17171,#17172);
#15405=AXIS2_PLACEMENT_3D('',#21117,#17173,#17174);
#15406=AXIS2_PLACEMENT_3D('',#21120,#17176,#17177);
#15407=AXIS2_PLACEMENT_3D('',#21121,#17178,#17179);
#15408=AXIS2_PLACEMENT_3D('',#21130,#17184,#17185);
#15409=AXIS2_PLACEMENT_3D('',#21133,#17187,#17188);
#15410=AXIS2_PLACEMENT_3D('',#21134,#17189,#17190);
#15411=AXIS2_PLACEMENT_3D('',#21137,#17192,#17193);
#15412=AXIS2_PLACEMENT_3D('',#21138,#17194,#17195);
#15413=AXIS2_PLACEMENT_3D('',#21141,#17197,#17198);
#15414=AXIS2_PLACEMENT_3D('',#21142,#17199,#17200);
#15415=AXIS2_PLACEMENT_3D('',#21144,#17201,#17202);
#15416=AXIS2_PLACEMENT_3D('',#21145,#17203,#17204);
#15417=AXIS2_PLACEMENT_3D('',#21147,#17205,#17206);
#15418=AXIS2_PLACEMENT_3D('',#21148,#17207,#17208);
#15419=AXIS2_PLACEMENT_3D('',#21150,#17209,#17210);
#15420=AXIS2_PLACEMENT_3D('',#21151,#17211,#17212);
#15421=AXIS2_PLACEMENT_3D('',#21154,#17214,#17215);
#15422=AXIS2_PLACEMENT_3D('',#21155,#17216,#17217);
#15423=AXIS2_PLACEMENT_3D('',#21158,#17219,#17220);
#15424=AXIS2_PLACEMENT_3D('',#21159,#17221,#17222);
#15425=AXIS2_PLACEMENT_3D('',#21162,#17224,#17225);
#15426=AXIS2_PLACEMENT_3D('',#21163,#17226,#17227);
#15427=AXIS2_PLACEMENT_3D('',#21165,#17228,#17229);
#15428=AXIS2_PLACEMENT_3D('',#21168,#17231,#17232);
#15429=AXIS2_PLACEMENT_3D('',#21169,#17233,#17234);
#15430=AXIS2_PLACEMENT_3D('',#21199,#17249,#17250);
#15431=AXIS2_PLACEMENT_3D('',#21201,#17251,#17252);
#15432=AXIS2_PLACEMENT_3D('',#21203,#17253,#17254);
#15433=AXIS2_PLACEMENT_3D('',#21204,#17255,#17256);
#15434=AXIS2_PLACEMENT_3D('',#21208,#17258,#17259);
#15435=AXIS2_PLACEMENT_3D('',#21209,#17260,#17261);
#15436=AXIS2_PLACEMENT_3D('',#21210,#17262,#17263);
#15437=AXIS2_PLACEMENT_3D('',#21212,#17264,#17265);
#15438=AXIS2_PLACEMENT_3D('',#21214,#17267,#17268);
#15439=AXIS2_PLACEMENT_3D('',#21218,#17270,#17271);
#15440=AXIS2_PLACEMENT_3D('',#21219,#17272,#17273);
#15441=AXIS2_PLACEMENT_3D('',#21220,#17274,#17275);
#15442=AXIS2_PLACEMENT_3D('',#21222,#17276,#17277);
#15443=AXIS2_PLACEMENT_3D('',#21224,#17279,#17280);
#15444=AXIS2_PLACEMENT_3D('',#21228,#17282,#17283);
#15445=AXIS2_PLACEMENT_3D('',#21229,#17284,#17285);
#15446=AXIS2_PLACEMENT_3D('',#21230,#17286,#17287);
#15447=AXIS2_PLACEMENT_3D('',#21232,#17288,#17289);
#15448=AXIS2_PLACEMENT_3D('',#21234,#17291,#17292);
#15449=AXIS2_PLACEMENT_3D('',#21238,#17294,#17295);
#15450=AXIS2_PLACEMENT_3D('',#21239,#17296,#17297);
#15451=AXIS2_PLACEMENT_3D('',#21240,#17298,#17299);
#15452=AXIS2_PLACEMENT_3D('',#21243,#17301,#17302);
#15453=AXIS2_PLACEMENT_3D('',#21246,#17304,#17305);
#15454=AXIS2_PLACEMENT_3D('',#21249,#17307,#17308);
#15455=AXIS2_PLACEMENT_3D('',#21252,#17310,#17311);
#15456=AXIS2_PLACEMENT_3D('',#21254,#17312,#17313);
#15457=AXIS2_PLACEMENT_3D('',#21257,#17315,#17316);
#15458=AXIS2_PLACEMENT_3D('',#21258,#17317,#17318);
#15459=AXIS2_PLACEMENT_3D('',#21288,#17333,#17334);
#15460=AXIS2_PLACEMENT_3D('',#21290,#17335,#17336);
#15461=AXIS2_PLACEMENT_3D('',#21292,#17337,#17338);
#15462=AXIS2_PLACEMENT_3D('',#21293,#17339,#17340);
#15463=AXIS2_PLACEMENT_3D('',#21297,#17342,#17343);
#15464=AXIS2_PLACEMENT_3D('',#21298,#17344,#17345);
#15465=AXIS2_PLACEMENT_3D('',#21299,#17346,#17347);
#15466=AXIS2_PLACEMENT_3D('',#21301,#17348,#17349);
#15467=AXIS2_PLACEMENT_3D('',#21303,#17351,#17352);
#15468=AXIS2_PLACEMENT_3D('',#21307,#17354,#17355);
#15469=AXIS2_PLACEMENT_3D('',#21308,#17356,#17357);
#15470=AXIS2_PLACEMENT_3D('',#21309,#17358,#17359);
#15471=AXIS2_PLACEMENT_3D('',#21311,#17360,#17361);
#15472=AXIS2_PLACEMENT_3D('',#21313,#17363,#17364);
#15473=AXIS2_PLACEMENT_3D('',#21317,#17366,#17367);
#15474=AXIS2_PLACEMENT_3D('',#21318,#17368,#17369);
#15475=AXIS2_PLACEMENT_3D('',#21319,#17370,#17371);
#15476=AXIS2_PLACEMENT_3D('',#21321,#17372,#17373);
#15477=AXIS2_PLACEMENT_3D('',#21323,#17375,#17376);
#15478=AXIS2_PLACEMENT_3D('',#21327,#17378,#17379);
#15479=AXIS2_PLACEMENT_3D('',#21328,#17380,#17381);
#15480=AXIS2_PLACEMENT_3D('',#21329,#17382,#17383);
#15481=AXIS2_PLACEMENT_3D('',#21332,#17385,#17386);
#15482=AXIS2_PLACEMENT_3D('',#21335,#17388,#17389);
#15483=AXIS2_PLACEMENT_3D('',#21338,#17391,#17392);
#15484=AXIS2_PLACEMENT_3D('',#21341,#17394,#17395);
#15485=AXIS2_PLACEMENT_3D('',#21343,#17396,#17397);
#15486=AXIS2_PLACEMENT_3D('',#21346,#17399,#17400);
#15487=AXIS2_PLACEMENT_3D('',#21347,#17401,#17402);
#15488=AXIS2_PLACEMENT_3D('',#21357,#17407,#17408);
#15489=AXIS2_PLACEMENT_3D('',#21359,#17409,#17410);
#15490=AXIS2_PLACEMENT_3D('',#21361,#17411,#17412);
#15491=AXIS2_PLACEMENT_3D('',#21363,#17413,#17414);
#15492=AXIS2_PLACEMENT_3D('',#21365,#17415,#17416);
#15493=AXIS2_PLACEMENT_3D('',#21367,#17417,#17418);
#15494=AXIS2_PLACEMENT_3D('',#21369,#17419,#17420);
#15495=AXIS2_PLACEMENT_3D('',#21371,#17421,#17422);
#15496=AXIS2_PLACEMENT_3D('',#21373,#17423,#17424);
#15497=AXIS2_PLACEMENT_3D('',#21375,#17425,#17426);
#15498=AXIS2_PLACEMENT_3D('',#21377,#17427,#17428);
#15499=AXIS2_PLACEMENT_3D('',#21379,#17429,#17430);
#15500=AXIS2_PLACEMENT_3D('',#21381,#17431,#17432);
#15501=AXIS2_PLACEMENT_3D('',#21382,#17433,#17434);
#15502=AXIS2_PLACEMENT_3D('',#21385,#17436,#17437);
#15503=AXIS2_PLACEMENT_3D('',#21386,#17438,#17439);
#15504=AXIS2_PLACEMENT_3D('',#21388,#17440,#17441);
#15505=AXIS2_PLACEMENT_3D('',#21390,#17443,#17444);
#15506=AXIS2_PLACEMENT_3D('',#21393,#17446,#17447);
#15507=AXIS2_PLACEMENT_3D('',#21394,#17448,#17449);
#15508=AXIS2_PLACEMENT_3D('',#21396,#17450,#17451);
#15509=AXIS2_PLACEMENT_3D('',#21398,#17453,#17454);
#15510=AXIS2_PLACEMENT_3D('',#21401,#17456,#17457);
#15511=AXIS2_PLACEMENT_3D('',#21402,#17458,#17459);
#15512=AXIS2_PLACEMENT_3D('',#21404,#17460,#17461);
#15513=AXIS2_PLACEMENT_3D('',#21406,#17463,#17464);
#15514=AXIS2_PLACEMENT_3D('',#21409,#17466,#17467);
#15515=AXIS2_PLACEMENT_3D('',#21410,#17468,#17469);
#15516=AXIS2_PLACEMENT_3D('',#21412,#17470,#17471);
#15517=AXIS2_PLACEMENT_3D('',#21414,#17473,#17474);
#15518=AXIS2_PLACEMENT_3D('',#21417,#17476,#17477);
#15519=AXIS2_PLACEMENT_3D('',#21418,#17478,#17479);
#15520=AXIS2_PLACEMENT_3D('',#21420,#17480,#17481);
#15521=AXIS2_PLACEMENT_3D('',#21422,#17483,#17484);
#15522=AXIS2_PLACEMENT_3D('',#21425,#17486,#17487);
#15523=AXIS2_PLACEMENT_3D('',#21426,#17488,#17489);
#15524=AXIS2_PLACEMENT_3D('',#21429,#17491,#17492);
#15525=AXIS2_PLACEMENT_3D('',#21432,#17494,#17495);
#15526=AXIS2_PLACEMENT_3D('',#21435,#17497,#17498);
#15527=AXIS2_PLACEMENT_3D('',#21438,#17500,#17501);
#15528=AXIS2_PLACEMENT_3D('',#21441,#17503,#17504);
#15529=AXIS2_PLACEMENT_3D('',#21444,#17506,#17507);
#15530=AXIS2_PLACEMENT_3D('',#21446,#17508,#17509);
#15531=AXIS2_PLACEMENT_3D('',#21448,#17511,#17512);
#15532=AXIS2_PLACEMENT_3D('',#21451,#17514,#17515);
#15533=AXIS2_PLACEMENT_3D('',#21452,#17516,#17517);
#15534=AXIS2_PLACEMENT_3D('',#21454,#17518,#17519);
#15535=AXIS2_PLACEMENT_3D('',#21456,#17521,#17522);
#15536=AXIS2_PLACEMENT_3D('',#21459,#17524,#17525);
#15537=AXIS2_PLACEMENT_3D('',#21460,#17526,#17527);
#15538=AXIS2_PLACEMENT_3D('',#21462,#17528,#17529);
#15539=AXIS2_PLACEMENT_3D('',#21464,#17531,#17532);
#15540=AXIS2_PLACEMENT_3D('',#21467,#17534,#17535);
#15541=AXIS2_PLACEMENT_3D('',#21468,#17536,#17537);
#15542=AXIS2_PLACEMENT_3D('',#21470,#17538,#17539);
#15543=AXIS2_PLACEMENT_3D('',#21472,#17541,#17542);
#15544=AXIS2_PLACEMENT_3D('',#21475,#17544,#17545);
#15545=AXIS2_PLACEMENT_3D('',#21476,#17546,#17547);
#15546=AXIS2_PLACEMENT_3D('',#21478,#17548,#17549);
#15547=AXIS2_PLACEMENT_3D('',#21480,#17551,#17552);
#15548=AXIS2_PLACEMENT_3D('',#21483,#17554,#17555);
#15549=AXIS2_PLACEMENT_3D('',#21484,#17556,#17557);
#15550=AXIS2_PLACEMENT_3D('',#21486,#17558,#17559);
#15551=AXIS2_PLACEMENT_3D('',#21488,#17561,#17562);
#15552=AXIS2_PLACEMENT_3D('',#21491,#17564,#17565);
#15553=AXIS2_PLACEMENT_3D('',#21492,#17566,#17567);
#15554=AXIS2_PLACEMENT_3D('',#21494,#17568,#17569);
#15555=AXIS2_PLACEMENT_3D('',#21496,#17571,#17572);
#15556=AXIS2_PLACEMENT_3D('',#21499,#17574,#17575);
#15557=AXIS2_PLACEMENT_3D('',#21500,#17576,#17577);
#15558=AXIS2_PLACEMENT_3D('',#21502,#17578,#17579);
#15559=AXIS2_PLACEMENT_3D('',#21504,#17581,#17582);
#15560=AXIS2_PLACEMENT_3D('',#21507,#17584,#17585);
#15561=AXIS2_PLACEMENT_3D('',#21508,#17586,#17587);
#15562=AXIS2_PLACEMENT_3D('',#21510,#17588,#17589);
#15563=AXIS2_PLACEMENT_3D('',#21511,#17590,#17591);
#15564=AXIS2_PLACEMENT_3D('',#21513,#17592,#17593);
#15565=AXIS2_PLACEMENT_3D('',#21514,#17594,#17595);
#15566=AXIS2_PLACEMENT_3D('',#21516,#17596,#17597);
#15567=AXIS2_PLACEMENT_3D('',#21517,#17598,#17599);
#15568=AXIS2_PLACEMENT_3D('',#21519,#17600,#17601);
#15569=AXIS2_PLACEMENT_3D('',#21520,#17602,#17603);
#15570=AXIS2_PLACEMENT_3D('',#21522,#17604,#17605);
#15571=AXIS2_PLACEMENT_3D('',#21523,#17606,#17607);
#15572=AXIS2_PLACEMENT_3D('',#21525,#17608,#17609);
#15573=AXIS2_PLACEMENT_3D('',#21526,#17610,#17611);
#15574=AXIS2_PLACEMENT_3D('',#21528,#17612,#17613);
#15575=AXIS2_PLACEMENT_3D('',#21529,#17614,#17615);
#15576=AXIS2_PLACEMENT_3D('',#21531,#17616,#17617);
#15577=AXIS2_PLACEMENT_3D('',#21532,#17618,#17619);
#15578=AXIS2_PLACEMENT_3D('',#21535,#17621,#17622);
#15579=AXIS2_PLACEMENT_3D('',#21536,#17623,#17624);
#15580=AXIS2_PLACEMENT_3D('',#21539,#17626,#17627);
#15581=AXIS2_PLACEMENT_3D('',#21540,#17628,#17629);
#15582=AXIS2_PLACEMENT_3D('',#21543,#17631,#17632);
#15583=AXIS2_PLACEMENT_3D('',#21544,#17633,#17634);
#15584=AXIS2_PLACEMENT_3D('',#21547,#17636,#17637);
#15585=AXIS2_PLACEMENT_3D('',#21548,#17638,#17639);
#15586=AXIS2_PLACEMENT_3D('',#21551,#17641,#17642);
#15587=AXIS2_PLACEMENT_3D('',#21552,#17643,#17644);
#15588=AXIS2_PLACEMENT_3D('',#21555,#17646,#17647);
#15589=AXIS2_PLACEMENT_3D('',#21556,#17648,#17649);
#15590=AXIS2_PLACEMENT_3D('',#21559,#17651,#17652);
#15591=AXIS2_PLACEMENT_3D('',#21560,#17653,#17654);
#15592=AXIS2_PLACEMENT_3D('',#21563,#17656,#17657);
#15593=AXIS2_PLACEMENT_3D('',#21564,#17658,#17659);
#15594=AXIS2_PLACEMENT_3D('',#21569,#17663,#17664);
#15595=AXIS2_PLACEMENT_3D('',#21574,#17668,#17669);
#15596=AXIS2_PLACEMENT_3D('',#21577,#17672,#17673);
#15597=AXIS2_PLACEMENT_3D('',#21582,#17677,#17678);
#15598=AXIS2_PLACEMENT_3D('',#21584,#17680,#17681);
#15599=AXIS2_PLACEMENT_3D('',#21587,#17684,#17685);
#15600=AXIS2_PLACEMENT_3D('',#21591,#17688,#17689);
#15601=AXIS2_PLACEMENT_3D('',#21593,#17691,#17692);
#15602=AXIS2_PLACEMENT_3D('',#21594,#17693,#17694);
#15603=AXIS2_PLACEMENT_3D('',#21597,#17697,#17698);
#15604=AXIS2_PLACEMENT_3D('',#21599,#17700,#17701);
#15605=AXIS2_PLACEMENT_3D('',#21602,#17704,#17705);
#15606=AXIS2_PLACEMENT_3D('',#21604,#17707,#17708);
#15607=AXIS2_PLACEMENT_3D('',#21605,#17709,#17710);
#15608=AXIS2_PLACEMENT_3D('',#21606,#17711,#17712);
#15609=AXIS2_PLACEMENT_3D('',#21608,#17714,#17715);
#15610=AXIS2_PLACEMENT_3D('',#21610,#17717,#17718);
#15611=AXIS2_PLACEMENT_3D('',#21612,#17720,#17721);
#15612=AXIS2_PLACEMENT_3D('',#21614,#17723,#17724);
#15613=AXIS2_PLACEMENT_3D('',#21616,#17726,#17727);
#16990=DIRECTION('axis',(0.,0.,1.));
#16991=DIRECTION('refdir',(1.,0.,0.));
#16992=DIRECTION('center_axis',(0.,0.,1.));
#16993=DIRECTION('ref_axis',(1.,0.,0.));
#16994=DIRECTION('center_axis',(0.,0.,-1.));
#16995=DIRECTION('ref_axis',(1.,0.,0.));
#16996=DIRECTION('',(-0.707106781186547,-8.65956056235493E-17,0.707106781186548));
#16997=DIRECTION('center_axis',(0.,0.,1.));
#16998=DIRECTION('ref_axis',(1.,0.,0.));
#16999=DIRECTION('center_axis',(0.,0.,1.));
#17000=DIRECTION('ref_axis',(1.,0.,0.));
#17001=DIRECTION('center_axis',(0.,0.,1.));
#17002=DIRECTION('ref_axis',(1.,0.,0.));
#17003=DIRECTION('center_axis',(0.,0.,-1.));
#17004=DIRECTION('ref_axis',(1.,0.,0.));
#17005=DIRECTION('',(-0.707106781186569,-8.65956056235519E-17,0.707106781186526));
#17006=DIRECTION('center_axis',(0.,0.,1.));
#17007=DIRECTION('ref_axis',(1.,0.,0.));
#17008=DIRECTION('center_axis',(0.,0.,1.));
#17009=DIRECTION('ref_axis',(1.,0.,0.));
#17010=DIRECTION('center_axis',(0.,0.,-1.));
#17011=DIRECTION('ref_axis',(1.,0.,0.));
#17012=DIRECTION('',(0.,0.,-1.));
#17013=DIRECTION('center_axis',(0.,0.,1.));
#17014=DIRECTION('ref_axis',(1.,0.,0.));
#17015=DIRECTION('center_axis',(0.,0.,1.));
#17016=DIRECTION('ref_axis',(1.,0.,0.));
#17017=DIRECTION('center_axis',(0.,0.,-1.));
#17018=DIRECTION('ref_axis',(1.,0.,0.));
#17019=DIRECTION('',(-0.707106781186547,-8.65956056235493E-17,0.707106781186548));
#17020=DIRECTION('center_axis',(0.,0.,1.));
#17021=DIRECTION('ref_axis',(1.,0.,0.));
#17022=DIRECTION('center_axis',(0.,0.,1.));
#17023=DIRECTION('ref_axis',(1.,0.,0.));
#17024=DIRECTION('center_axis',(0.,0.,1.));
#17025=DIRECTION('ref_axis',(1.,0.,0.));
#17026=DIRECTION('center_axis',(0.,0.,-1.));
#17027=DIRECTION('ref_axis',(1.,0.,0.));
#17028=DIRECTION('',(-0.707106781186547,-8.65956056235493E-17,0.707106781186548));
#17029=DIRECTION('center_axis',(0.,0.,1.));
#17030=DIRECTION('ref_axis',(1.,0.,0.));
#17031=DIRECTION('center_axis',(0.,0.,1.));
#17032=DIRECTION('ref_axis',(1.,0.,0.));
#17033=DIRECTION('center_axis',(0.,0.,-1.));
#17034=DIRECTION('ref_axis',(1.,0.,0.));
#17035=DIRECTION('',(0.,0.,-1.));
#17036=DIRECTION('center_axis',(0.,0.,1.));
#17037=DIRECTION('ref_axis',(1.,0.,0.));
#17038=DIRECTION('center_axis',(0.,0.,1.));
#17039=DIRECTION('ref_axis',(1.,0.,0.));
#17040=DIRECTION('center_axis',(0.,0.,-1.));
#17041=DIRECTION('ref_axis',(1.,0.,0.));
#17042=DIRECTION('',(-0.707106781186558,-8.65956056235506E-17,0.707106781186537));
#17043=DIRECTION('center_axis',(0.,0.,1.));
#17044=DIRECTION('ref_axis',(1.,0.,0.));
#17045=DIRECTION('center_axis',(0.,0.,1.));
#17046=DIRECTION('ref_axis',(1.,0.,0.));
#17047=DIRECTION('center_axis',(0.,0.,1.));
#17048=DIRECTION('ref_axis',(1.,0.,0.));
#17049=DIRECTION('center_axis',(0.,0.,-1.));
#17050=DIRECTION('ref_axis',(1.,0.,0.));
#17051=DIRECTION('',(-0.707106781186558,-8.65956056235506E-17,0.707106781186537));
#17052=DIRECTION('center_axis',(0.,0.,1.));
#17053=DIRECTION('ref_axis',(1.,0.,0.));
#17054=DIRECTION('center_axis',(0.,0.,1.));
#17055=DIRECTION('ref_axis',(1.,0.,0.));
#17056=DIRECTION('center_axis',(0.,0.,-1.));
#17057=DIRECTION('ref_axis',(1.,0.,0.));
#17058=DIRECTION('',(0.,0.,-1.));
#17059=DIRECTION('center_axis',(0.,0.,1.));
#17060=DIRECTION('ref_axis',(1.,0.,0.));
#17061=DIRECTION('center_axis',(0.,0.,1.));
#17062=DIRECTION('ref_axis',(0.,-1.,0.));
#17063=DIRECTION('',(0.,-1.,0.));
#17064=DIRECTION('',(1.,0.,0.));
#17065=DIRECTION('',(0.,1.,0.));
#17066=DIRECTION('',(-1.,0.,0.));
#17067=DIRECTION('center_axis',(0.,0.,-1.));
#17068=DIRECTION('ref_axis',(1.,0.,0.));
#17069=DIRECTION('',(0.,0.,-1.));
#17070=DIRECTION('center_axis',(0.,0.,-1.));
#17071=DIRECTION('ref_axis',(1.,0.,0.));
#17072=DIRECTION('center_axis',(0.,0.,-1.));
#17073=DIRECTION('ref_axis',(1.,0.,0.));
#17074=DIRECTION('',(0.,0.,-1.));
#17075=DIRECTION('center_axis',(0.,0.,-1.));
#17076=DIRECTION('ref_axis',(1.,0.,0.));
#17077=DIRECTION('center_axis',(0.,0.,-1.));
#17078=DIRECTION('ref_axis',(1.,0.,0.));
#17079=DIRECTION('',(0.,0.,-1.));
#17080=DIRECTION('center_axis',(0.,0.,-1.));
#17081=DIRECTION('ref_axis',(1.,0.,0.));
#17082=DIRECTION('center_axis',(0.,0.,1.));
#17083=DIRECTION('ref_axis',(1.,0.,0.));
#17084=DIRECTION('center_axis',(0.,0.,1.));
#17085=DIRECTION('ref_axis',(1.,0.,0.));
#17086=DIRECTION('center_axis',(0.,0.,1.));
#17087=DIRECTION('ref_axis',(1.,0.,0.));
#17088=DIRECTION('center_axis',(0.,0.,1.));
#17089=DIRECTION('ref_axis',(1.,0.,0.));
#17090=DIRECTION('center_axis',(0.,0.,1.));
#17091=DIRECTION('ref_axis',(1.,0.,0.));
#17092=DIRECTION('center_axis',(0.,0.,1.));
#17093=DIRECTION('ref_axis',(1.,0.,0.));
#17094=DIRECTION('center_axis',(0.,0.,-1.));
#17095=DIRECTION('ref_axis',(1.,0.,0.));
#17096=DIRECTION('',(0.,0.,-1.));
#17097=DIRECTION('center_axis',(0.,0.,1.));
#17098=DIRECTION('ref_axis',(1.,0.,0.));
#17099=DIRECTION('center_axis',(0.,0.,-1.));
#17100=DIRECTION('ref_axis',(1.,0.,0.));
#17101=DIRECTION('',(0.,0.,-1.));
#17102=DIRECTION('center_axis',(0.,0.,1.));
#17103=DIRECTION('ref_axis',(1.,0.,0.));
#17104=DIRECTION('center_axis',(0.,0.,-1.));
#17105=DIRECTION('ref_axis',(1.,0.,0.));
#17106=DIRECTION('',(0.,0.,-1.));
#17107=DIRECTION('center_axis',(0.,0.,1.));
#17108=DIRECTION('ref_axis',(1.,0.,0.));
#17109=DIRECTION('center_axis',(0.,0.,-1.));
#17110=DIRECTION('ref_axis',(1.,0.,0.));
#17111=DIRECTION('center_axis',(0.,0.,1.));
#17112=DIRECTION('ref_axis',(1.,0.,0.));
#17113=DIRECTION('',(-0.70710678118654,8.65956056235484E-17,-0.707106781186555));
#17114=DIRECTION('center_axis',(0.,0.,-1.));
#17115=DIRECTION('ref_axis',(1.,0.,0.));
#17116=DIRECTION('center_axis',(0.,0.,-1.));
#17117=DIRECTION('ref_axis',(1.,0.,0.));
#17118=DIRECTION('center_axis',(0.,0.,-1.));
#17119=DIRECTION('ref_axis',(1.,0.,0.));
#17120=DIRECTION('center_axis',(0.,0.,1.));
#17121=DIRECTION('ref_axis',(1.,0.,0.));
#17122=DIRECTION('',(-0.707106781186561,8.6595605623551E-17,-0.707106781186534));
#17123=DIRECTION('center_axis',(0.,0.,-1.));
#17124=DIRECTION('ref_axis',(1.,0.,0.));
#17125=DIRECTION('center_axis',(0.,0.,-1.));
#17126=DIRECTION('ref_axis',(1.,0.,0.));
#17127=DIRECTION('center_axis',(0.,0.,1.));
#17128=DIRECTION('ref_axis',(1.,0.,0.));
#17129=DIRECTION('',(0.,0.,1.));
#17130=DIRECTION('center_axis',(0.,0.,-1.));
#17131=DIRECTION('ref_axis',(1.,0.,0.));
#17132=DIRECTION('center_axis',(0.,0.,-1.));
#17133=DIRECTION('ref_axis',(1.,0.,0.));
#17134=DIRECTION('center_axis',(0.,0.,1.));
#17135=DIRECTION('ref_axis',(1.,0.,0.));
#17136=DIRECTION('',(-0.70710678118654,8.65956056235484E-17,-0.707106781186555));
#17137=DIRECTION('center_axis',(0.,0.,-1.));
#17138=DIRECTION('ref_axis',(1.,0.,0.));
#17139=DIRECTION('center_axis',(0.,0.,-1.));
#17140=DIRECTION('ref_axis',(1.,0.,0.));
#17141=DIRECTION('center_axis',(0.,0.,-1.));
#17142=DIRECTION('ref_axis',(1.,0.,0.));
#17143=DIRECTION('center_axis',(0.,0.,1.));
#17144=DIRECTION('ref_axis',(1.,0.,0.));
#17145=DIRECTION('',(-0.70710678118654,8.65956056235484E-17,-0.707106781186555));
#17146=DIRECTION('center_axis',(0.,0.,-1.));
#17147=DIRECTION('ref_axis',(1.,0.,0.));
#17148=DIRECTION('center_axis',(0.,0.,-1.));
#17149=DIRECTION('ref_axis',(1.,0.,0.));
#17150=DIRECTION('center_axis',(0.,0.,1.));
#17151=DIRECTION('ref_axis',(1.,0.,0.));
#17152=DIRECTION('',(0.,0.,1.));
#17153=DIRECTION('center_axis',(0.,0.,-1.));
#17154=DIRECTION('ref_axis',(1.,0.,0.));
#17155=DIRECTION('center_axis',(0.,0.,-1.));
#17156=DIRECTION('ref_axis',(1.,0.,0.));
#17157=DIRECTION('center_axis',(0.,0.,1.));
#17158=DIRECTION('ref_axis',(1.,0.,0.));
#17159=DIRECTION('',(-0.70710678118655,8.65956056235497E-17,-0.707106781186545));
#17160=DIRECTION('center_axis',(0.,0.,-1.));
#17161=DIRECTION('ref_axis',(1.,0.,0.));
#17162=DIRECTION('center_axis',(0.,0.,-1.));
#17163=DIRECTION('ref_axis',(1.,0.,0.));
#17164=DIRECTION('center_axis',(0.,0.,-1.));
#17165=DIRECTION('ref_axis',(1.,0.,0.));
#17166=DIRECTION('center_axis',(0.,0.,1.));
#17167=DIRECTION('ref_axis',(1.,0.,0.));
#17168=DIRECTION('',(-0.70710678118655,8.65956056235496E-17,-0.707106781186545));
#17169=DIRECTION('center_axis',(0.,0.,-1.));
#17170=DIRECTION('ref_axis',(1.,0.,0.));
#17171=DIRECTION('center_axis',(0.,0.,-1.));
#17172=DIRECTION('ref_axis',(1.,0.,0.));
#17173=DIRECTION('center_axis',(0.,0.,1.));
#17174=DIRECTION('ref_axis',(1.,0.,0.));
#17175=DIRECTION('',(0.,0.,1.));
#17176=DIRECTION('center_axis',(0.,0.,-1.));
#17177=DIRECTION('ref_axis',(1.,0.,0.));
#17178=DIRECTION('center_axis',(0.,0.,-1.));
#17179=DIRECTION('ref_axis',(0.,1.,0.));
#17180=DIRECTION('',(0.,1.,0.));
#17181=DIRECTION('',(1.,0.,0.));
#17182=DIRECTION('',(0.,-1.,0.));
#17183=DIRECTION('',(-1.,0.,0.));
#17184=DIRECTION('center_axis',(0.,0.,1.));
#17185=DIRECTION('ref_axis',(1.,0.,0.));
#17186=DIRECTION('',(0.,0.,1.));
#17187=DIRECTION('center_axis',(0.,0.,1.));
#17188=DIRECTION('ref_axis',(1.,0.,0.));
#17189=DIRECTION('center_axis',(0.,0.,1.));
#17190=DIRECTION('ref_axis',(1.,0.,0.));
#17191=DIRECTION('',(0.,0.,1.));
#17192=DIRECTION('center_axis',(0.,0.,1.));
#17193=DIRECTION('ref_axis',(1.,0.,0.));
#17194=DIRECTION('center_axis',(0.,0.,1.));
#17195=DIRECTION('ref_axis',(1.,0.,0.));
#17196=DIRECTION('',(0.,0.,1.));
#17197=DIRECTION('center_axis',(0.,0.,1.));
#17198=DIRECTION('ref_axis',(1.,0.,0.));
#17199=DIRECTION('center_axis',(0.,0.,1.));
#17200=DIRECTION('ref_axis',(1.,0.,0.));
#17201=DIRECTION('center_axis',(0.,0.,-1.));
#17202=DIRECTION('ref_axis',(1.,0.,0.));
#17203=DIRECTION('center_axis',(0.,0.,1.));
#17204=DIRECTION('ref_axis',(1.,0.,0.));
#17205=DIRECTION('center_axis',(0.,0.,-1.));
#17206=DIRECTION('ref_axis',(1.,0.,0.));
#17207=DIRECTION('center_axis',(0.,0.,1.));
#17208=DIRECTION('ref_axis',(1.,0.,0.));
#17209=DIRECTION('center_axis',(0.,0.,-1.));
#17210=DIRECTION('ref_axis',(1.,0.,0.));
#17211=DIRECTION('center_axis',(0.,0.,1.));
#17212=DIRECTION('ref_axis',(1.,0.,0.));
#17213=DIRECTION('',(0.,0.,1.));
#17214=DIRECTION('center_axis',(0.,0.,-1.));
#17215=DIRECTION('ref_axis',(1.,0.,0.));
#17216=DIRECTION('center_axis',(0.,0.,1.));
#17217=DIRECTION('ref_axis',(1.,0.,0.));
#17218=DIRECTION('',(0.,0.,1.));
#17219=DIRECTION('center_axis',(0.,0.,-1.));
#17220=DIRECTION('ref_axis',(1.,0.,0.));
#17221=DIRECTION('center_axis',(0.,0.,1.));
#17222=DIRECTION('ref_axis',(1.,0.,0.));
#17223=DIRECTION('',(0.,0.,1.));
#17224=DIRECTION('center_axis',(0.,0.,-1.));
#17225=DIRECTION('ref_axis',(1.,0.,0.));
#17226=DIRECTION('center_axis',(1.,0.,0.));
#17227=DIRECTION('ref_axis',(0.,0.,-1.));
#17228=DIRECTION('center_axis',(-1.,0.,0.));
#17229=DIRECTION('ref_axis',(0.,0.,-1.));
#17230=DIRECTION('',(0.707106781186568,-8.65956056235468E-17,0.707106781186527));
#17231=DIRECTION('center_axis',(1.,0.,0.));
#17232=DIRECTION('ref_axis',(0.,0.,-1.));
#17233=DIRECTION('center_axis',(1.,0.,0.));
#17234=DIRECTION('ref_axis',(0.,0.,-1.));
#17235=DIRECTION('',(0.,1.,0.));
#17236=DIRECTION('',(0.,0.,-1.));
#17237=DIRECTION('',(0.,-0.707106781186547,0.707106781186547));
#17238=DIRECTION('',(0.,1.,0.));
#17239=DIRECTION('',(0.,0.,-1.));
#17240=DIRECTION('',(0.,-1.,0.));
#17241=DIRECTION('',(0.,0.,-1.));
#17242=DIRECTION('',(0.,1.,0.));
#17243=DIRECTION('',(0.,0.,-1.));
#17244=DIRECTION('',(0.,-1.,0.));
#17245=DIRECTION('',(0.,0.707106781186555,0.70710678118654));
#17246=DIRECTION('',(0.,0.,-1.));
#17247=DIRECTION('',(0.,-1.,0.));
#17248=DIRECTION('',(0.,0.,-1.));
#17249=DIRECTION('center_axis',(1.,0.,0.));
#17250=DIRECTION('ref_axis',(0.,0.,-1.));
#17251=DIRECTION('center_axis',(1.,0.,0.));
#17252=DIRECTION('ref_axis',(0.,0.,-1.));
#17253=DIRECTION('center_axis',(1.,0.,0.));
#17254=DIRECTION('ref_axis',(0.,0.,-1.));
#17255=DIRECTION('center_axis',(-1.,0.,0.));
#17256=DIRECTION('ref_axis',(0.,0.,-1.));
#17257=DIRECTION('',(-1.,0.,0.));
#17258=DIRECTION('center_axis',(-1.,0.,0.));
#17259=DIRECTION('ref_axis',(0.,0.,-1.));
#17260=DIRECTION('center_axis',(-1.,0.,0.));
#17261=DIRECTION('ref_axis',(0.,0.,-1.));
#17262=DIRECTION('center_axis',(1.,0.,0.));
#17263=DIRECTION('ref_axis',(0.,0.,-1.));
#17264=DIRECTION('center_axis',(-1.,0.,0.));
#17265=DIRECTION('ref_axis',(0.,0.,-1.));
#17266=DIRECTION('',(0.70710678118656,-8.65956056235478E-17,0.707106781186535));
#17267=DIRECTION('center_axis',(-1.,0.,0.));
#17268=DIRECTION('ref_axis',(0.,0.,-1.));
#17269=DIRECTION('',(-1.,0.,0.));
#17270=DIRECTION('center_axis',(-1.,0.,0.));
#17271=DIRECTION('ref_axis',(0.,0.,-1.));
#17272=DIRECTION('center_axis',(-1.,0.,0.));
#17273=DIRECTION('ref_axis',(0.,0.,-1.));
#17274=DIRECTION('center_axis',(1.,0.,0.));
#17275=DIRECTION('ref_axis',(0.,0.,-1.));
#17276=DIRECTION('center_axis',(-1.,0.,0.));
#17277=DIRECTION('ref_axis',(0.,0.,-1.));
#17278=DIRECTION('',(0.707106781186558,-8.65956056235481E-17,0.707106781186537));
#17279=DIRECTION('center_axis',(-1.,0.,0.));
#17280=DIRECTION('ref_axis',(0.,0.,-1.));
#17281=DIRECTION('',(-1.,0.,0.));
#17282=DIRECTION('center_axis',(-1.,0.,0.));
#17283=DIRECTION('ref_axis',(0.,0.,-1.));
#17284=DIRECTION('center_axis',(-1.,0.,0.));
#17285=DIRECTION('ref_axis',(0.,0.,-1.));
#17286=DIRECTION('center_axis',(1.,0.,0.));
#17287=DIRECTION('ref_axis',(0.,0.,-1.));
#17288=DIRECTION('center_axis',(-1.,0.,0.));
#17289=DIRECTION('ref_axis',(0.,0.,-1.));
#17290=DIRECTION('',(0.707106781186561,-8.65956056235477E-17,0.707106781186534));
#17291=DIRECTION('center_axis',(-1.,0.,0.));
#17292=DIRECTION('ref_axis',(0.,0.,-1.));
#17293=DIRECTION('',(-1.,0.,0.));
#17294=DIRECTION('center_axis',(-1.,0.,0.));
#17295=DIRECTION('ref_axis',(0.,0.,-1.));
#17296=DIRECTION('center_axis',(-1.,0.,0.));
#17297=DIRECTION('ref_axis',(0.,0.,-1.));
#17298=DIRECTION('center_axis',(1.,0.,0.));
#17299=DIRECTION('ref_axis',(0.,1.,0.));
#17300=DIRECTION('',(0.515038074910049,-0.857167300702115,-1.04972719113862E-16));
#17301=DIRECTION('center_axis',(1.,0.,0.));
#17302=DIRECTION('ref_axis',(0.,1.,0.));
#17303=DIRECTION('',(0.515038074910049,-0.857167300702115,-1.04972719113862E-16));
#17304=DIRECTION('center_axis',(1.,0.,0.));
#17305=DIRECTION('ref_axis',(0.,1.,0.));
#17306=DIRECTION('',(0.515038074910049,-0.857167300702115,-1.04972719113862E-16));
#17307=DIRECTION('center_axis',(1.,0.,0.));
#17308=DIRECTION('ref_axis',(0.,1.,0.));
#17309=DIRECTION('',(0.515038074910049,-0.857167300702115,-1.04972719113862E-16));
#17310=DIRECTION('center_axis',(-1.,0.,0.));
#17311=DIRECTION('ref_axis',(0.,0.,-1.));
#17312=DIRECTION('center_axis',(1.,0.,0.));
#17313=DIRECTION('ref_axis',(0.,0.,-1.));
#17314=DIRECTION('',(-0.707106781186555,8.65956056235485E-17,0.70710678118654));
#17315=DIRECTION('center_axis',(-1.,0.,0.));
#17316=DIRECTION('ref_axis',(0.,0.,-1.));
#17317=DIRECTION('center_axis',(1.,0.,0.));
#17318=DIRECTION('ref_axis',(0.,0.,-1.));
#17319=DIRECTION('',(0.,1.,0.));
#17320=DIRECTION('',(0.,0.,-1.));
#17321=DIRECTION('',(0.,-0.707106781186555,-0.70710678118654));
#17322=DIRECTION('',(0.,-1.,0.));
#17323=DIRECTION('',(0.,0.,-1.));
#17324=DIRECTION('',(0.,1.,0.));
#17325=DIRECTION('',(0.,0.,-1.));
#17326=DIRECTION('',(0.,-1.,0.));
#17327=DIRECTION('',(0.,0.,-1.));
#17328=DIRECTION('',(0.,1.,0.));
#17329=DIRECTION('',(0.,0.707106781186547,-0.707106781186547));
#17330=DIRECTION('',(0.,0.,-1.));
#17331=DIRECTION('',(0.,-1.,0.));
#17332=DIRECTION('',(0.,0.,1.));
#17333=DIRECTION('center_axis',(-1.,0.,0.));
#17334=DIRECTION('ref_axis',(0.,0.,-1.));
#17335=DIRECTION('center_axis',(-1.,0.,0.));
#17336=DIRECTION('ref_axis',(0.,0.,-1.));
#17337=DIRECTION('center_axis',(-1.,0.,0.));
#17338=DIRECTION('ref_axis',(0.,0.,-1.));
#17339=DIRECTION('center_axis',(1.,0.,0.));
#17340=DIRECTION('ref_axis',(0.,0.,-1.));
#17341=DIRECTION('',(1.,0.,0.));
#17342=DIRECTION('center_axis',(1.,0.,0.));
#17343=DIRECTION('ref_axis',(0.,0.,-1.));
#17344=DIRECTION('center_axis',(1.,0.,0.));
#17345=DIRECTION('ref_axis',(0.,0.,-1.));
#17346=DIRECTION('center_axis',(-1.,0.,0.));
#17347=DIRECTION('ref_axis',(0.,0.,-1.));
#17348=DIRECTION('center_axis',(1.,0.,0.));
#17349=DIRECTION('ref_axis',(0.,0.,-1.));
#17350=DIRECTION('',(-0.707106781186547,8.65956056235494E-17,0.707106781186548));
#17351=DIRECTION('center_axis',(1.,0.,0.));
#17352=DIRECTION('ref_axis',(0.,0.,-1.));
#17353=DIRECTION('',(1.,0.,0.));
#17354=DIRECTION('center_axis',(1.,0.,0.));
#17355=DIRECTION('ref_axis',(0.,0.,-1.));
#17356=DIRECTION('center_axis',(1.,0.,0.));
#17357=DIRECTION('ref_axis',(0.,0.,-1.));
#17358=DIRECTION('center_axis',(-1.,0.,0.));
#17359=DIRECTION('ref_axis',(0.,0.,-1.));
#17360=DIRECTION('center_axis',(1.,0.,0.));
#17361=DIRECTION('ref_axis',(0.,0.,-1.));
#17362=DIRECTION('',(-0.707106781186545,8.65956056235496E-17,0.70710678118655));
#17363=DIRECTION('center_axis',(1.,0.,0.));
#17364=DIRECTION('ref_axis',(0.,0.,-1.));
#17365=DIRECTION('',(1.,0.,0.));
#17366=DIRECTION('center_axis',(1.,0.,0.));
#17367=DIRECTION('ref_axis',(0.,0.,-1.));
#17368=DIRECTION('center_axis',(1.,0.,0.));
#17369=DIRECTION('ref_axis',(0.,0.,-1.));
#17370=DIRECTION('center_axis',(-1.,0.,0.));
#17371=DIRECTION('ref_axis',(0.,0.,-1.));
#17372=DIRECTION('center_axis',(1.,0.,0.));
#17373=DIRECTION('ref_axis',(0.,0.,-1.));
#17374=DIRECTION('',(-0.707106781186548,8.65956056235493E-17,0.707106781186547));
#17375=DIRECTION('center_axis',(1.,0.,0.));
#17376=DIRECTION('ref_axis',(0.,0.,-1.));
#17377=DIRECTION('',(1.,0.,0.));
#17378=DIRECTION('center_axis',(1.,0.,0.));
#17379=DIRECTION('ref_axis',(0.,0.,-1.));
#17380=DIRECTION('center_axis',(1.,0.,0.));
#17381=DIRECTION('ref_axis',(0.,0.,-1.));
#17382=DIRECTION('center_axis',(-1.,0.,0.));
#17383=DIRECTION('ref_axis',(0.,1.,0.));
#17384=DIRECTION('',(-0.515038074910058,-0.85716730070211,1.04972719113862E-16));
#17385=DIRECTION('center_axis',(-1.,0.,0.));
#17386=DIRECTION('ref_axis',(0.,1.,0.));
#17387=DIRECTION('',(-0.515038074910058,-0.85716730070211,1.04972719113862E-16));
#17388=DIRECTION('center_axis',(-1.,0.,0.));
#17389=DIRECTION('ref_axis',(0.,1.,0.));
#17390=DIRECTION('',(-0.515038074910058,-0.85716730070211,1.04972719113862E-16));
#17391=DIRECTION('center_axis',(-1.,0.,0.));
#17392=DIRECTION('ref_axis',(0.,1.,0.));
#17393=DIRECTION('',(-0.515038074910058,-0.85716730070211,1.04972719113862E-16));
#17394=DIRECTION('center_axis',(0.,1.,0.));
#17395=DIRECTION('ref_axis',(1.,0.,0.));
#17396=DIRECTION('center_axis',(0.,-1.,0.));
#17397=DIRECTION('ref_axis',(1.,0.,0.));
#17398=DIRECTION('',(-0.707106781186539,0.707106781186555,8.65956056235483E-17));
#17399=DIRECTION('center_axis',(0.,1.,0.));
#17400=DIRECTION('ref_axis',(1.,0.,0.));
#17401=DIRECTION('center_axis',(0.,1.,0.));
#17402=DIRECTION('ref_axis',(0.,0.,1.));
#17403=DIRECTION('',(0.,0.,1.));
#17404=DIRECTION('',(1.,0.,0.));
#17405=DIRECTION('',(0.,0.,-1.));
#17406=DIRECTION('',(-1.,0.,0.));
#17407=DIRECTION('center_axis',(0.,1.,0.));
#17408=DIRECTION('ref_axis',(1.,0.,0.));
#17409=DIRECTION('center_axis',(0.,1.,0.));
#17410=DIRECTION('ref_axis',(1.,0.,0.));
#17411=DIRECTION('center_axis',(0.,1.,0.));
#17412=DIRECTION('ref_axis',(1.,0.,0.));
#17413=DIRECTION('center_axis',(0.,1.,0.));
#17414=DIRECTION('ref_axis',(1.,0.,0.));
#17415=DIRECTION('center_axis',(0.,1.,0.));
#17416=DIRECTION('ref_axis',(1.,0.,0.));
#17417=DIRECTION('center_axis',(0.,1.,0.));
#17418=DIRECTION('ref_axis',(1.,0.,0.));
#17419=DIRECTION('center_axis',(0.,1.,0.));
#17420=DIRECTION('ref_axis',(1.,0.,0.));
#17421=DIRECTION('center_axis',(0.,1.,0.));
#17422=DIRECTION('ref_axis',(1.,0.,0.));
#17423=DIRECTION('center_axis',(0.,1.,0.));
#17424=DIRECTION('ref_axis',(1.,0.,0.));
#17425=DIRECTION('center_axis',(0.,1.,0.));
#17426=DIRECTION('ref_axis',(1.,0.,0.));
#17427=DIRECTION('center_axis',(0.,1.,0.));
#17428=DIRECTION('ref_axis',(1.,0.,0.));
#17429=DIRECTION('center_axis',(0.,1.,0.));
#17430=DIRECTION('ref_axis',(1.,0.,0.));
#17431=DIRECTION('center_axis',(0.,1.,0.));
#17432=DIRECTION('ref_axis',(1.,0.,0.));
#17433=DIRECTION('center_axis',(0.,-1.,0.));
#17434=DIRECTION('ref_axis',(1.,0.,0.));
#17435=DIRECTION('',(0.,-1.,0.));
#17436=DIRECTION('center_axis',(0.,-1.,0.));
#17437=DIRECTION('ref_axis',(1.,0.,0.));
#17438=DIRECTION('center_axis',(0.,1.,0.));
#17439=DIRECTION('ref_axis',(1.,0.,0.));
#17440=DIRECTION('center_axis',(0.,-1.,0.));
#17441=DIRECTION('ref_axis',(1.,0.,0.));
#17442=DIRECTION('',(-0.707106781186539,0.707106781186555,8.65956056235483E-17));
#17443=DIRECTION('center_axis',(0.,-1.,0.));
#17444=DIRECTION('ref_axis',(1.,0.,0.));
#17445=DIRECTION('',(0.,-1.,0.));
#17446=DIRECTION('center_axis',(0.,-1.,0.));
#17447=DIRECTION('ref_axis',(1.,0.,0.));
#17448=DIRECTION('center_axis',(0.,1.,0.));
#17449=DIRECTION('ref_axis',(1.,0.,0.));
#17450=DIRECTION('center_axis',(0.,-1.,0.));
#17451=DIRECTION('ref_axis',(1.,0.,0.));
#17452=DIRECTION('',(-0.707106781186539,0.707106781186555,8.65956056235483E-17));
#17453=DIRECTION('center_axis',(0.,-1.,0.));
#17454=DIRECTION('ref_axis',(1.,0.,0.));
#17455=DIRECTION('',(0.,-1.,0.));
#17456=DIRECTION('center_axis',(0.,-1.,0.));
#17457=DIRECTION('ref_axis',(1.,0.,0.));
#17458=DIRECTION('center_axis',(0.,1.,0.));
#17459=DIRECTION('ref_axis',(1.,0.,0.));
#17460=DIRECTION('center_axis',(0.,-1.,0.));
#17461=DIRECTION('ref_axis',(1.,0.,0.));
#17462=DIRECTION('',(-0.707106781186547,0.707106781186548,8.65956056235493E-17));
#17463=DIRECTION('center_axis',(0.,-1.,0.));
#17464=DIRECTION('ref_axis',(1.,0.,0.));
#17465=DIRECTION('',(0.,-1.,0.));
#17466=DIRECTION('center_axis',(0.,-1.,0.));
#17467=DIRECTION('ref_axis',(1.,0.,0.));
#17468=DIRECTION('center_axis',(0.,1.,0.));
#17469=DIRECTION('ref_axis',(1.,0.,0.));
#17470=DIRECTION('center_axis',(0.,-1.,0.));
#17471=DIRECTION('ref_axis',(1.,0.,0.));
#17472=DIRECTION('',(-0.707106781186547,0.707106781186548,8.65956056235493E-17));
#17473=DIRECTION('center_axis',(0.,-1.,0.));
#17474=DIRECTION('ref_axis',(1.,0.,0.));
#17475=DIRECTION('',(0.,-1.,0.));
#17476=DIRECTION('center_axis',(0.,-1.,0.));
#17477=DIRECTION('ref_axis',(1.,0.,0.));
#17478=DIRECTION('center_axis',(0.,1.,0.));
#17479=DIRECTION('ref_axis',(1.,0.,0.));
#17480=DIRECTION('center_axis',(0.,-1.,0.));
#17481=DIRECTION('ref_axis',(1.,0.,0.));
#17482=DIRECTION('',(-0.707106781186539,0.707106781186555,8.65956056235483E-17));
#17483=DIRECTION('center_axis',(0.,-1.,0.));
#17484=DIRECTION('ref_axis',(1.,0.,0.));
#17485=DIRECTION('',(0.,-1.,0.));
#17486=DIRECTION('center_axis',(0.,-1.,0.));
#17487=DIRECTION('ref_axis',(1.,0.,0.));
#17488=DIRECTION('center_axis',(0.,1.,0.));
#17489=DIRECTION('ref_axis',(1.,0.,0.));
#17490=DIRECTION('',(-0.857167300702115,0.515038074910049,1.04972719113862E-16));
#17491=DIRECTION('center_axis',(0.,1.,0.));
#17492=DIRECTION('ref_axis',(1.,0.,0.));
#17493=DIRECTION('',(-0.857167300702115,0.515038074910049,1.04972719113862E-16));
#17494=DIRECTION('center_axis',(0.,1.,0.));
#17495=DIRECTION('ref_axis',(1.,0.,0.));
#17496=DIRECTION('',(-0.85716730070211,0.515038074910058,1.04972719113862E-16));
#17497=DIRECTION('center_axis',(0.,1.,0.));
#17498=DIRECTION('ref_axis',(1.,0.,0.));
#17499=DIRECTION('',(-0.85716730070211,0.515038074910058,1.04972719113862E-16));
#17500=DIRECTION('center_axis',(0.,1.,0.));
#17501=DIRECTION('ref_axis',(1.,0.,0.));
#17502=DIRECTION('',(-0.85716730070211,0.515038074910058,1.04972719113862E-16));
#17503=DIRECTION('center_axis',(0.,1.,0.));
#17504=DIRECTION('ref_axis',(1.,0.,0.));
#17505=DIRECTION('',(-0.85716730070211,0.515038074910058,1.04972719113862E-16));
#17506=DIRECTION('center_axis',(0.,1.,0.));
#17507=DIRECTION('ref_axis',(1.,0.,0.));
#17508=DIRECTION('center_axis',(0.,-1.,0.));
#17509=DIRECTION('ref_axis',(1.,0.,0.));
#17510=DIRECTION('',(-0.707106781186558,0.707106781186537,8.65956056235506E-17));
#17511=DIRECTION('center_axis',(0.,-1.,0.));
#17512=DIRECTION('ref_axis',(1.,0.,0.));
#17513=DIRECTION('',(0.,-1.,0.));
#17514=DIRECTION('center_axis',(0.,-1.,0.));
#17515=DIRECTION('ref_axis',(1.,0.,0.));
#17516=DIRECTION('center_axis',(0.,1.,0.));
#17517=DIRECTION('ref_axis',(1.,0.,0.));
#17518=DIRECTION('center_axis',(0.,-1.,0.));
#17519=DIRECTION('ref_axis',(1.,0.,0.));
#17520=DIRECTION('',(-0.707106781186537,0.707106781186558,8.65956056235481E-17));
#17521=DIRECTION('center_axis',(0.,-1.,0.));
#17522=DIRECTION('ref_axis',(1.,0.,0.));
#17523=DIRECTION('',(0.,-1.,0.));
#17524=DIRECTION('center_axis',(0.,-1.,0.));
#17525=DIRECTION('ref_axis',(1.,0.,0.));
#17526=DIRECTION('center_axis',(0.,1.,0.));
#17527=DIRECTION('ref_axis',(1.,0.,0.));
#17528=DIRECTION('center_axis',(0.,-1.,0.));
#17529=DIRECTION('ref_axis',(1.,0.,0.));
#17530=DIRECTION('',(-0.707106781186542,0.707106781186553,8.65956056235487E-17));
#17531=DIRECTION('center_axis',(0.,-1.,0.));
#17532=DIRECTION('ref_axis',(1.,0.,0.));
#17533=DIRECTION('',(0.,-1.,0.));
#17534=DIRECTION('center_axis',(0.,-1.,0.));
#17535=DIRECTION('ref_axis',(1.,0.,0.));
#17536=DIRECTION('center_axis',(0.,1.,0.));
#17537=DIRECTION('ref_axis',(1.,0.,0.));
#17538=DIRECTION('center_axis',(0.,-1.,0.));
#17539=DIRECTION('ref_axis',(1.,0.,0.));
#17540=DIRECTION('',(-0.707106781186537,0.707106781186558,8.65956056235481E-17));
#17541=DIRECTION('center_axis',(0.,-1.,0.));
#17542=DIRECTION('ref_axis',(1.,0.,0.));
#17543=DIRECTION('',(0.,-1.,0.));
#17544=DIRECTION('center_axis',(0.,-1.,0.));
#17545=DIRECTION('ref_axis',(1.,0.,0.));
#17546=DIRECTION('center_axis',(0.,1.,0.));
#17547=DIRECTION('ref_axis',(1.,0.,0.));
#17548=DIRECTION('center_axis',(0.,-1.,0.));
#17549=DIRECTION('ref_axis',(1.,0.,0.));
#17550=DIRECTION('',(-0.707106781186542,0.707106781186553,8.65956056235487E-17));
#17551=DIRECTION('center_axis',(0.,-1.,0.));
#17552=DIRECTION('ref_axis',(1.,0.,0.));
#17553=DIRECTION('',(0.,-1.,0.));
#17554=DIRECTION('center_axis',(0.,-1.,0.));
#17555=DIRECTION('ref_axis',(1.,0.,0.));
#17556=DIRECTION('center_axis',(0.,1.,0.));
#17557=DIRECTION('ref_axis',(1.,0.,0.));
#17558=DIRECTION('center_axis',(0.,-1.,0.));
#17559=DIRECTION('ref_axis',(1.,0.,0.));
#17560=DIRECTION('',(-0.707106781186537,0.707106781186558,8.65956056235481E-17));
#17561=DIRECTION('center_axis',(0.,-1.,0.));
#17562=DIRECTION('ref_axis',(1.,0.,0.));
#17563=DIRECTION('',(0.,-1.,0.));
#17564=DIRECTION('center_axis',(0.,-1.,0.));
#17565=DIRECTION('ref_axis',(1.,0.,0.));
#17566=DIRECTION('center_axis',(0.,1.,0.));
#17567=DIRECTION('ref_axis',(1.,0.,0.));
#17568=DIRECTION('center_axis',(0.,-1.,0.));
#17569=DIRECTION('ref_axis',(1.,0.,0.));
#17570=DIRECTION('',(-0.707106781186537,0.707106781186558,8.65956056235481E-17));
#17571=DIRECTION('center_axis',(0.,-1.,0.));
#17572=DIRECTION('ref_axis',(1.,0.,0.));
#17573=DIRECTION('',(0.,-1.,0.));
#17574=DIRECTION('center_axis',(0.,-1.,0.));
#17575=DIRECTION('ref_axis',(1.,0.,0.));
#17576=DIRECTION('center_axis',(0.,1.,0.));
#17577=DIRECTION('ref_axis',(1.,0.,0.));
#17578=DIRECTION('center_axis',(0.,-1.,0.));
#17579=DIRECTION('ref_axis',(1.,0.,0.));
#17580=DIRECTION('',(-0.707106781186558,0.707106781186537,8.65956056235506E-17));
#17581=DIRECTION('center_axis',(0.,-1.,0.));
#17582=DIRECTION('ref_axis',(1.,0.,0.));
#17583=DIRECTION('',(0.,-1.,0.));
#17584=DIRECTION('center_axis',(0.,-1.,0.));
#17585=DIRECTION('ref_axis',(1.,0.,0.));
#17586=DIRECTION('center_axis',(0.,1.,0.));
#17587=DIRECTION('ref_axis',(1.,0.,0.));
#17588=DIRECTION('center_axis',(0.,1.,0.));
#17589=DIRECTION('ref_axis',(1.,0.,0.));
#17590=DIRECTION('center_axis',(0.,1.,0.));
#17591=DIRECTION('ref_axis',(1.,0.,0.));
#17592=DIRECTION('center_axis',(0.,1.,0.));
#17593=DIRECTION('ref_axis',(1.,0.,0.));
#17594=DIRECTION('center_axis',(0.,1.,0.));
#17595=DIRECTION('ref_axis',(1.,0.,0.));
#17596=DIRECTION('center_axis',(0.,1.,0.));
#17597=DIRECTION('ref_axis',(1.,0.,0.));
#17598=DIRECTION('center_axis',(0.,1.,0.));
#17599=DIRECTION('ref_axis',(1.,0.,0.));
#17600=DIRECTION('center_axis',(0.,1.,0.));
#17601=DIRECTION('ref_axis',(1.,0.,0.));
#17602=DIRECTION('center_axis',(0.,1.,0.));
#17603=DIRECTION('ref_axis',(1.,0.,0.));
#17604=DIRECTION('center_axis',(0.,1.,0.));
#17605=DIRECTION('ref_axis',(1.,0.,0.));
#17606=DIRECTION('center_axis',(0.,1.,0.));
#17607=DIRECTION('ref_axis',(1.,0.,0.));
#17608=DIRECTION('center_axis',(0.,1.,0.));
#17609=DIRECTION('ref_axis',(1.,0.,0.));
#17610=DIRECTION('center_axis',(0.,1.,0.));
#17611=DIRECTION('ref_axis',(1.,0.,0.));
#17612=DIRECTION('center_axis',(0.,1.,0.));
#17613=DIRECTION('ref_axis',(1.,0.,0.));
#17614=DIRECTION('center_axis',(0.,1.,0.));
#17615=DIRECTION('ref_axis',(1.,0.,0.));
#17616=DIRECTION('center_axis',(0.,1.,0.));
#17617=DIRECTION('ref_axis',(1.,0.,0.));
#17618=DIRECTION('center_axis',(0.,-1.,0.));
#17619=DIRECTION('ref_axis',(1.,0.,0.));
#17620=DIRECTION('',(0.,-1.,0.));
#17621=DIRECTION('center_axis',(0.,1.,0.));
#17622=DIRECTION('ref_axis',(1.,0.,0.));
#17623=DIRECTION('center_axis',(0.,-1.,0.));
#17624=DIRECTION('ref_axis',(1.,0.,0.));
#17625=DIRECTION('',(0.,-1.,0.));
#17626=DIRECTION('center_axis',(0.,1.,0.));
#17627=DIRECTION('ref_axis',(1.,0.,0.));
#17628=DIRECTION('center_axis',(0.,-1.,0.));
#17629=DIRECTION('ref_axis',(1.,0.,0.));
#17630=DIRECTION('',(0.,-1.,0.));
#17631=DIRECTION('center_axis',(0.,1.,0.));
#17632=DIRECTION('ref_axis',(1.,0.,0.));
#17633=DIRECTION('center_axis',(0.,-1.,0.));
#17634=DIRECTION('ref_axis',(1.,0.,0.));
#17635=DIRECTION('',(0.,-1.,0.));
#17636=DIRECTION('center_axis',(0.,1.,0.));
#17637=DIRECTION('ref_axis',(1.,0.,0.));
#17638=DIRECTION('center_axis',(0.,-1.,0.));
#17639=DIRECTION('ref_axis',(1.,0.,0.));
#17640=DIRECTION('',(0.,-1.,0.));
#17641=DIRECTION('center_axis',(0.,1.,0.));
#17642=DIRECTION('ref_axis',(1.,0.,0.));
#17643=DIRECTION('center_axis',(0.,-1.,0.));
#17644=DIRECTION('ref_axis',(1.,0.,0.));
#17645=DIRECTION('',(0.,-1.,0.));
#17646=DIRECTION('center_axis',(0.,1.,0.));
#17647=DIRECTION('ref_axis',(1.,0.,0.));
#17648=DIRECTION('center_axis',(0.,-1.,0.));
#17649=DIRECTION('ref_axis',(1.,0.,0.));
#17650=DIRECTION('',(0.,-1.,0.));
#17651=DIRECTION('center_axis',(0.,1.,0.));
#17652=DIRECTION('ref_axis',(1.,0.,0.));
#17653=DIRECTION('center_axis',(0.,-1.,0.));
#17654=DIRECTION('ref_axis',(1.,0.,0.));
#17655=DIRECTION('',(0.,-1.,0.));
#17656=DIRECTION('center_axis',(0.,1.,0.));
#17657=DIRECTION('ref_axis',(1.,0.,0.));
#17658=DIRECTION('center_axis',(0.707106781186548,0.,0.707106781186548));
#17659=DIRECTION('ref_axis',(0.707106781186548,0.,-0.707106781186548));
#17660=DIRECTION('',(0.577350269189628,-0.577350269189621,-0.577350269189628));
#17661=DIRECTION('',(-0.577350269189629,0.577350269189619,0.577350269189629));
#17662=DIRECTION('',(-0.577350269189626,-0.577350269189626,0.577350269189626));
#17663=DIRECTION('center_axis',(0.707106781186541,0.707106781186554,0.));
#17664=DIRECTION('ref_axis',(0.,0.,-1.));
#17665=DIRECTION('',(-0.577350269189633,0.577350269189622,-0.577350269189622));
#17666=DIRECTION('',(-0.577350269189632,0.577350269189622,0.577350269189624));
#17667=DIRECTION('',(0.577350269189633,-0.577350269189622,0.577350269189622));
#17668=DIRECTION('center_axis',(0.,-0.707106781186552,0.707106781186543));
#17669=DIRECTION('ref_axis',(1.,0.,0.));
#17670=DIRECTION('',(0.577350269189623,0.577350269189623,0.577350269189631));
#17671=DIRECTION('',(1.,0.,0.));
#17672=DIRECTION('center_axis',(0.,0.707106781186549,-0.707106781186546));
#17673=DIRECTION('ref_axis',(-1.,0.,0.));
#17674=DIRECTION('',(0.577350269189633,0.577350269189621,0.577350269189623));
#17675=DIRECTION('',(0.577350269189628,-0.577350269189624,-0.577350269189626));
#17676=DIRECTION('',(-0.577350269189627,-0.577350269189624,-0.577350269189627));
#17677=DIRECTION('center_axis',(0.707106781186541,0.,-0.707106781186554));
#17678=DIRECTION('ref_axis',(-0.707106781186554,0.,-0.707106781186541));
#17679=DIRECTION('',(-0.577350269189634,0.577350269189621,-0.577350269189623));
#17680=DIRECTION('center_axis',(-0.707106781186546,0.,-0.707106781186549));
#17681=DIRECTION('ref_axis',(-0.707106781186549,0.,0.707106781186546));
#17682=DIRECTION('',(-0.577350269189628,-0.577350269189623,0.577350269189626));
#17683=DIRECTION('',(0.577350269189627,0.577350269189625,-0.577350269189625));
#17684=DIRECTION('center_axis',(-0.707106781186546,0.707106781186549,0.));
#17685=DIRECTION('ref_axis',(0.,0.,1.));
#17686=DIRECTION('',(0.577350269189624,0.577350269189622,0.577350269189632));
#17687=DIRECTION('',(0.577350269189627,0.577350269189625,-0.577350269189625));
#17688=DIRECTION('center_axis',(0.,0.707106781186548,0.707106781186548));
#17689=DIRECTION('ref_axis',(1.,0.,0.));
#17690=DIRECTION('',(-0.57735026918962,0.577350269189629,-0.577350269189629));
#17691=DIRECTION('center_axis',(-0.707106781186553,0.,0.707106781186543));
#17692=DIRECTION('ref_axis',(0.707106781186543,0.,0.707106781186553));
#17693=DIRECTION('center_axis',(0.,-0.70710678118654,0.707106781186555));
#17694=DIRECTION('ref_axis',(1.,0.,0.));
#17695=DIRECTION('',(-1.,0.,0.));
#17696=DIRECTION('',(1.,0.,0.));
#17697=DIRECTION('center_axis',(0.,-1.,0.));
#17698=DIRECTION('ref_axis',(0.,0.,-1.));
#17699=DIRECTION('',(-1.,0.,0.));
#17700=DIRECTION('center_axis',(0.,-0.707106781186548,-0.707106781186548));
#17701=DIRECTION('ref_axis',(-1.,0.,0.));
#17702=DIRECTION('',(-1.,0.,0.));
#17703=DIRECTION('',(1.,0.,0.));
#17704=DIRECTION('center_axis',(0.,0.,-1.));
#17705=DIRECTION('ref_axis',(0.,1.,0.));
#17706=DIRECTION('',(1.,0.,0.));
#17707=DIRECTION('center_axis',(0.,-0.707106781186549,-0.707106781186546));
#17708=DIRECTION('ref_axis',(-1.,0.,0.));
#17709=DIRECTION('center_axis',(0.,-1.,0.));
#17710=DIRECTION('ref_axis',(0.,0.,-1.));
#17711=DIRECTION('center_axis',(0.,0.,1.));
#17712=DIRECTION('ref_axis',(0.,-1.,0.));
#17713=DIRECTION('',(1.,0.,0.));
#17714=DIRECTION('center_axis',(0.,-1.,0.));
#17715=DIRECTION('ref_axis',(0.,0.,-1.));
#17716=DIRECTION('',(1.,0.,0.));
#17717=DIRECTION('center_axis',(0.,0.,-1.));
#17718=DIRECTION('ref_axis',(0.,1.,0.));
#17719=DIRECTION('',(1.,0.,0.));
#17720=DIRECTION('center_axis',(0.,-1.,0.));
#17721=DIRECTION('ref_axis',(0.,0.,-1.));
#17722=DIRECTION('',(1.,0.,0.));
#17723=DIRECTION('center_axis',(0.,0.,1.));
#17724=DIRECTION('ref_axis',(0.,-1.,0.));
#17725=DIRECTION('',(1.,0.,0.));
#17726=DIRECTION('center_axis',(0.,-1.,0.));
#17727=DIRECTION('ref_axis',(0.,0.,-1.));
#20922=CARTESIAN_POINT('',(0.,0.,0.));
#20923=CARTESIAN_POINT('Origin',(155.,29.,99.85));
#20924=CARTESIAN_POINT('',(152.45,29.,99.7));
#20925=CARTESIAN_POINT('Origin',(155.,29.,99.7));
#20926=CARTESIAN_POINT('',(152.15,29.,100.));
#20927=CARTESIAN_POINT('',(152.3,29.,99.85));
#20928=CARTESIAN_POINT('',(154.259173435261,26.24796875,100.));
#20929=CARTESIAN_POINT('Origin',(155.,29.,100.));
#20930=CARTESIAN_POINT('',(155.740826564739,26.24796875,100.));
#20931=CARTESIAN_POINT('Ctrl Pts',(154.259173435261,26.24796875,99.9999999999999));
#20932=CARTESIAN_POINT('Ctrl Pts',(154.508665267946,26.2326405180042,99.9499486302178));
#20933=CARTESIAN_POINT('Ctrl Pts',(154.758456056481,26.225,99.925));
#20934=CARTESIAN_POINT('Ctrl Pts',(155.241543943519,26.225,99.925));
#20935=CARTESIAN_POINT('Ctrl Pts',(155.491334732054,26.2326405180042,99.9499486302178));
#20936=CARTESIAN_POINT('Ctrl Pts',(155.740826564739,26.24796875,99.9999999999999));
#20937=CARTESIAN_POINT('Origin',(155.,29.,100.));
#20938=CARTESIAN_POINT('Origin',(155.,21.,99.85));
#20939=CARTESIAN_POINT('',(150.,21.,99.7));
#20940=CARTESIAN_POINT('Origin',(155.,21.,99.7));
#20941=CARTESIAN_POINT('',(149.7,21.,100.));
#20942=CARTESIAN_POINT('',(149.85,21.,99.85));
#20943=CARTESIAN_POINT('Origin',(155.,21.,100.));
#20944=CARTESIAN_POINT('Origin',(155.,21.,100.));
#20945=CARTESIAN_POINT('Origin',(155.,29.,100.));
#20946=CARTESIAN_POINT('',(152.45,29.,75.5));
#20947=CARTESIAN_POINT('',(152.45,29.,100.));
#20948=CARTESIAN_POINT('Origin',(155.,29.,75.5));
#20949=CARTESIAN_POINT('Origin',(105.,29.,99.85));
#20950=CARTESIAN_POINT('',(102.45,29.,99.7));
#20951=CARTESIAN_POINT('Origin',(105.,29.,99.7));
#20952=CARTESIAN_POINT('',(102.15,29.,100.));
#20953=CARTESIAN_POINT('',(102.3,29.,99.85));
#20954=CARTESIAN_POINT('',(104.259173435261,26.24796875,100.));
#20955=CARTESIAN_POINT('Origin',(105.,29.,100.));
#20956=CARTESIAN_POINT('',(105.740826564739,26.24796875,100.));
#20957=CARTESIAN_POINT('Ctrl Pts',(104.259173435261,26.24796875,99.9999999999999));
#20958=CARTESIAN_POINT('Ctrl Pts',(104.508665267946,26.2326405180042,99.9499486302178));
#20959=CARTESIAN_POINT('Ctrl Pts',(104.758456056481,26.225,99.925));
#20960=CARTESIAN_POINT('Ctrl Pts',(105.241543943519,26.225,99.925));
#20961=CARTESIAN_POINT('Ctrl Pts',(105.491334732054,26.2326405180042,99.9499486302178));
#20962=CARTESIAN_POINT('Ctrl Pts',(105.740826564739,26.24796875,99.9999999999999));
#20963=CARTESIAN_POINT('Origin',(105.,29.,100.));
#20964=CARTESIAN_POINT('Origin',(105.,21.,99.85));
#20965=CARTESIAN_POINT('',(100.,21.,99.7));
#20966=CARTESIAN_POINT('Origin',(105.,21.,99.7));
#20967=CARTESIAN_POINT('',(99.7,21.,100.));
#20968=CARTESIAN_POINT('',(99.85,21.,99.85));
#20969=CARTESIAN_POINT('Origin',(105.,21.,100.));
#20970=CARTESIAN_POINT('Origin',(105.,21.,100.));
#20971=CARTESIAN_POINT('Origin',(105.,29.,100.));
#20972=CARTESIAN_POINT('',(102.45,29.,75.5));
#20973=CARTESIAN_POINT('',(102.45,29.,100.));
#20974=CARTESIAN_POINT('Origin',(105.,29.,75.5));
#20975=CARTESIAN_POINT('Origin',(55.,29.,99.85));
#20976=CARTESIAN_POINT('',(52.45,29.,99.7));
#20977=CARTESIAN_POINT('Origin',(55.,29.,99.7));
#20978=CARTESIAN_POINT('',(52.15,29.,100.));
#20979=CARTESIAN_POINT('',(52.3,29.,99.85));
#20980=CARTESIAN_POINT('',(54.2591734352607,26.24796875,100.));
#20981=CARTESIAN_POINT('Origin',(55.,29.,100.));
#20982=CARTESIAN_POINT('',(55.7408265647393,26.24796875,100.));
#20983=CARTESIAN_POINT('Ctrl Pts',(54.2591734352607,26.24796875,100.));
#20984=CARTESIAN_POINT('Ctrl Pts',(54.5086652679461,26.2326405180042,99.9499486302178));
#20985=CARTESIAN_POINT('Ctrl Pts',(54.7584560564804,26.225,99.925));
#20986=CARTESIAN_POINT('Ctrl Pts',(55.2415439435196,26.225,99.925));
#20987=CARTESIAN_POINT('Ctrl Pts',(55.4913347320539,26.2326405180042,99.9499486302178));
#20988=CARTESIAN_POINT('Ctrl Pts',(55.7408265647393,26.24796875,100.));
#20989=CARTESIAN_POINT('Origin',(55.,29.,100.));
#20990=CARTESIAN_POINT('Origin',(55.,21.,99.85));
#20991=CARTESIAN_POINT('',(50.,21.,99.7));
#20992=CARTESIAN_POINT('Origin',(55.,21.,99.7));
#20993=CARTESIAN_POINT('',(49.7,21.,100.));
#20994=CARTESIAN_POINT('',(49.85,21.,99.85));
#20995=CARTESIAN_POINT('Origin',(55.,21.,100.));
#20996=CARTESIAN_POINT('Origin',(55.,21.,100.));
#20997=CARTESIAN_POINT('Origin',(55.,29.,100.));
#20998=CARTESIAN_POINT('',(52.45,29.,75.5));
#20999=CARTESIAN_POINT('',(52.45,29.,100.));
#21000=CARTESIAN_POINT('Origin',(55.,29.,75.5));
#21001=CARTESIAN_POINT('Origin',(0.,45.,100.));
#21002=CARTESIAN_POINT('',(209.5,44.5,100.));
#21003=CARTESIAN_POINT('',(209.5,14.5,100.));
#21004=CARTESIAN_POINT('',(209.5,37.25,100.));
#21005=CARTESIAN_POINT('',(0.5,44.5,100.));
#21006=CARTESIAN_POINT('',(0.,44.5,100.));
#21007=CARTESIAN_POINT('',(0.5,14.5,100.));
#21008=CARTESIAN_POINT('',(0.5,37.25,100.));
#21009=CARTESIAN_POINT('',(0.,14.5,100.));
#21010=CARTESIAN_POINT('Origin',(155.,21.,100.));
#21011=CARTESIAN_POINT('',(150.,21.,92.5));
#21012=CARTESIAN_POINT('',(150.,21.,100.));
#21013=CARTESIAN_POINT('Origin',(155.,21.,92.5));
#21014=CARTESIAN_POINT('Origin',(105.,21.,100.));
#21015=CARTESIAN_POINT('',(100.,21.,92.5));
#21016=CARTESIAN_POINT('',(100.,21.,100.));
#21017=CARTESIAN_POINT('Origin',(105.,21.,92.5));
#21018=CARTESIAN_POINT('Origin',(55.,21.,100.));
#21019=CARTESIAN_POINT('',(50.,21.,92.5));
#21020=CARTESIAN_POINT('',(50.,21.,100.));
#21021=CARTESIAN_POINT('Origin',(55.,21.,92.5));
#21022=CARTESIAN_POINT('Origin',(55.,21.,92.5));
#21023=CARTESIAN_POINT('',(52.,21.,92.5));
#21024=CARTESIAN_POINT('Origin',(55.,21.,92.5));
#21025=CARTESIAN_POINT('Origin',(105.,21.,92.5));
#21026=CARTESIAN_POINT('',(102.,21.,92.5));
#21027=CARTESIAN_POINT('Origin',(105.,21.,92.5));
#21028=CARTESIAN_POINT('Origin',(155.,21.,92.5));
#21029=CARTESIAN_POINT('',(152.,21.,92.5));
#21030=CARTESIAN_POINT('Origin',(155.,21.,92.5));
#21031=CARTESIAN_POINT('Origin',(55.,21.,100.));
#21032=CARTESIAN_POINT('',(52.,21.,75.5));
#21033=CARTESIAN_POINT('',(52.,21.,100.));
#21034=CARTESIAN_POINT('Origin',(55.,21.,75.5));
#21035=CARTESIAN_POINT('Origin',(105.,21.,100.));
#21036=CARTESIAN_POINT('',(102.,21.,75.5));
#21037=CARTESIAN_POINT('',(102.,21.,100.));
#21038=CARTESIAN_POINT('Origin',(105.,21.,75.5));
#21039=CARTESIAN_POINT('Origin',(155.,21.,100.));
#21040=CARTESIAN_POINT('',(152.,21.,75.5));
#21041=CARTESIAN_POINT('',(152.,21.,100.));
#21042=CARTESIAN_POINT('Origin',(155.,21.,75.5));
#21043=CARTESIAN_POINT('Origin',(155.,29.,0.15));
#21044=CARTESIAN_POINT('',(152.45,29.,0.3));
#21045=CARTESIAN_POINT('Origin',(155.,29.,0.3));
#21046=CARTESIAN_POINT('',(152.15,29.,-4.59701721133854E-15));
#21047=CARTESIAN_POINT('',(152.3,29.,0.15));
#21048=CARTESIAN_POINT('',(155.740826564739,26.24796875,0.));
#21049=CARTESIAN_POINT('Origin',(155.,29.,0.));
#21050=CARTESIAN_POINT('',(154.259173435261,26.24796875,0.));
#21051=CARTESIAN_POINT('Ctrl Pts',(155.740826564739,26.24796875,6.73332917200398E-14));
#21052=CARTESIAN_POINT('Ctrl Pts',(155.491334732054,26.2326405180042,0.0500513697821895));
#21053=CARTESIAN_POINT('Ctrl Pts',(155.241543943519,26.225,0.0750000000000045));
#21054=CARTESIAN_POINT('Ctrl Pts',(154.758456056481,26.225,0.0750000000000045));
#21055=CARTESIAN_POINT('Ctrl Pts',(154.508665267946,26.2326405180042,0.0500513697821932));
#21056=CARTESIAN_POINT('Ctrl Pts',(154.259173435261,26.24796875,7.24507259741713E-14));
#21057=CARTESIAN_POINT('Origin',(155.,29.,0.));
#21058=CARTESIAN_POINT('Origin',(155.,21.,0.15));
#21059=CARTESIAN_POINT('',(150.,21.,0.3));
#21060=CARTESIAN_POINT('Origin',(155.,21.,0.3));
#21061=CARTESIAN_POINT('',(149.7,21.,-9.19403442267708E-15));
#21062=CARTESIAN_POINT('',(149.85,21.,0.15));
#21063=CARTESIAN_POINT('Origin',(155.,21.,0.));
#21064=CARTESIAN_POINT('Origin',(155.,21.,0.));
#21065=CARTESIAN_POINT('Origin',(155.,29.,0.));
#21066=CARTESIAN_POINT('',(152.45,29.,24.5));
#21067=CARTESIAN_POINT('',(152.45,29.,0.));
#21068=CARTESIAN_POINT('Origin',(155.,29.,24.5));
#21069=CARTESIAN_POINT('Origin',(105.,29.,0.15));
#21070=CARTESIAN_POINT('',(102.45,29.,0.3));
#21071=CARTESIAN_POINT('Origin',(105.,29.,0.3));
#21072=CARTESIAN_POINT('',(102.15,29.,-4.59701721133854E-15));
#21073=CARTESIAN_POINT('',(102.3,29.,0.15));
#21074=CARTESIAN_POINT('',(105.740826564739,26.24796875,0.));
#21075=CARTESIAN_POINT('Origin',(105.,29.,0.));
#21076=CARTESIAN_POINT('',(104.259173435261,26.24796875,0.));
#21077=CARTESIAN_POINT('Ctrl Pts',(105.740826564739,26.24796875,5.15299608538911E-14));
#21078=CARTESIAN_POINT('Ctrl Pts',(105.491334732054,26.2326405180042,0.0500513697821832));
#21079=CARTESIAN_POINT('Ctrl Pts',(105.241543943519,26.225,0.0749999999999978));
#21080=CARTESIAN_POINT('Ctrl Pts',(104.758456056481,26.225,0.0749999999999978));
#21081=CARTESIAN_POINT('Ctrl Pts',(104.508665267946,26.2326405180042,0.0500513697821799));
#21082=CARTESIAN_POINT('Ctrl Pts',(104.259173435261,26.24796875,5.67341312818215E-14));
#21083=CARTESIAN_POINT('Origin',(105.,29.,0.));
#21084=CARTESIAN_POINT('Origin',(105.,21.,0.15));
#21085=CARTESIAN_POINT('',(100.,21.,0.3));
#21086=CARTESIAN_POINT('Origin',(105.,21.,0.3));
#21087=CARTESIAN_POINT('',(99.7,21.,1.50920942409982E-15));
#21088=CARTESIAN_POINT('',(99.85,21.,0.15));
#21089=CARTESIAN_POINT('Origin',(105.,21.,0.));
#21090=CARTESIAN_POINT('Origin',(105.,21.,0.));
#21091=CARTESIAN_POINT('Origin',(105.,29.,0.));
#21092=CARTESIAN_POINT('',(102.45,29.,24.5));
#21093=CARTESIAN_POINT('',(102.45,29.,0.));
#21094=CARTESIAN_POINT('Origin',(105.,29.,24.5));
#21095=CARTESIAN_POINT('Origin',(55.,29.,0.15));
#21096=CARTESIAN_POINT('',(52.45,29.,0.3));
#21097=CARTESIAN_POINT('Origin',(55.,29.,0.3));
#21098=CARTESIAN_POINT('',(52.15,29.,-2.41126563160776E-15));
#21099=CARTESIAN_POINT('',(52.3,29.,0.15));
#21100=CARTESIAN_POINT('',(55.7408265647393,26.24796875,0.));
#21101=CARTESIAN_POINT('Origin',(55.,29.,0.));
#21102=CARTESIAN_POINT('',(54.2591734352607,26.24796875,0.));
#21103=CARTESIAN_POINT('Ctrl Pts',(55.7408265647393,26.24796875,-2.9316826744008E-15));
#21104=CARTESIAN_POINT('Ctrl Pts',(55.4913347320539,26.2326405180042,0.0500513697821647));
#21105=CARTESIAN_POINT('Ctrl Pts',(55.2415439435196,26.225,0.0749999999999999));
#21106=CARTESIAN_POINT('Ctrl Pts',(54.7584560564804,26.225,0.0749999999999999));
#21107=CARTESIAN_POINT('Ctrl Pts',(54.5086652679461,26.2326405180042,0.0500513697821644));
#21108=CARTESIAN_POINT('Ctrl Pts',(54.2591734352607,26.24796875,1.21430643318376E-15));
#21109=CARTESIAN_POINT('Origin',(55.,29.,0.));
#21110=CARTESIAN_POINT('Origin',(55.,21.,0.15));
#21111=CARTESIAN_POINT('',(50.,21.,0.3));
#21112=CARTESIAN_POINT('Origin',(55.,21.,0.3));
#21113=CARTESIAN_POINT('',(49.7,21.,-2.4980018054066E-15));
#21114=CARTESIAN_POINT('',(49.85,21.,0.15));
#21115=CARTESIAN_POINT('Origin',(55.,21.,0.));
#21116=CARTESIAN_POINT('Origin',(55.,21.,0.));
#21117=CARTESIAN_POINT('Origin',(55.,29.,0.));
#21118=CARTESIAN_POINT('',(52.45,29.,24.5));
#21119=CARTESIAN_POINT('',(52.45,29.,0.));
#21120=CARTESIAN_POINT('Origin',(55.,29.,24.5));
#21121=CARTESIAN_POINT('Origin',(0.,14.,0.));
#21122=CARTESIAN_POINT('',(209.5,14.5,0.));
#21123=CARTESIAN_POINT('',(209.5,44.5,0.));
#21124=CARTESIAN_POINT('',(209.5,21.75,0.));
#21125=CARTESIAN_POINT('',(0.5,14.5,0.));
#21126=CARTESIAN_POINT('',(0.,14.5,0.));
#21127=CARTESIAN_POINT('',(0.5,44.5,0.));
#21128=CARTESIAN_POINT('',(0.5,21.75,0.));
#21129=CARTESIAN_POINT('',(0.,44.5,0.));
#21130=CARTESIAN_POINT('Origin',(155.,21.,0.));
#21131=CARTESIAN_POINT('',(150.,21.,7.5));
#21132=CARTESIAN_POINT('',(150.,21.,0.));
#21133=CARTESIAN_POINT('Origin',(155.,21.,7.5));
#21134=CARTESIAN_POINT('Origin',(105.,21.,0.));
#21135=CARTESIAN_POINT('',(100.,21.,7.5));
#21136=CARTESIAN_POINT('',(100.,21.,0.));
#21137=CARTESIAN_POINT('Origin',(105.,21.,7.5));
#21138=CARTESIAN_POINT('Origin',(55.,21.,0.));
#21139=CARTESIAN_POINT('',(50.,21.,7.5));
#21140=CARTESIAN_POINT('',(50.,21.,0.));
#21141=CARTESIAN_POINT('Origin',(55.,21.,7.5));
#21142=CARTESIAN_POINT('Origin',(55.,21.,7.5));
#21143=CARTESIAN_POINT('',(52.,21.,7.5));
#21144=CARTESIAN_POINT('Origin',(55.,21.,7.5));
#21145=CARTESIAN_POINT('Origin',(105.,21.,7.5));
#21146=CARTESIAN_POINT('',(102.,21.,7.5));
#21147=CARTESIAN_POINT('Origin',(105.,21.,7.5));
#21148=CARTESIAN_POINT('Origin',(155.,21.,7.5));
#21149=CARTESIAN_POINT('',(152.,21.,7.5));
#21150=CARTESIAN_POINT('Origin',(155.,21.,7.5));
#21151=CARTESIAN_POINT('Origin',(55.,21.,0.));
#21152=CARTESIAN_POINT('',(52.,21.,24.5));
#21153=CARTESIAN_POINT('',(52.,21.,0.));
#21154=CARTESIAN_POINT('Origin',(55.,21.,24.5));
#21155=CARTESIAN_POINT('Origin',(105.,21.,0.));
#21156=CARTESIAN_POINT('',(102.,21.,24.5));
#21157=CARTESIAN_POINT('',(102.,21.,0.));
#21158=CARTESIAN_POINT('Origin',(105.,21.,24.5));
#21159=CARTESIAN_POINT('Origin',(155.,21.,0.));
#21160=CARTESIAN_POINT('',(152.,21.,24.5));
#21161=CARTESIAN_POINT('',(152.,21.,0.));
#21162=CARTESIAN_POINT('Origin',(155.,21.,24.5));
#21163=CARTESIAN_POINT('Origin',(209.85,30.,96.));
#21164=CARTESIAN_POINT('',(209.7,30.,98.05));
#21165=CARTESIAN_POINT('Origin',(209.7,30.,96.));
#21166=CARTESIAN_POINT('',(210.,30.,98.35));
#21167=CARTESIAN_POINT('',(209.85,30.,98.2));
#21168=CARTESIAN_POINT('Origin',(210.,30.,96.));
#21169=CARTESIAN_POINT('Origin',(210.,29.5,50.));
#21170=CARTESIAN_POINT('',(210.,14.,99.5));
#21171=CARTESIAN_POINT('',(210.,44.5,99.5));
#21172=CARTESIAN_POINT('',(210.,37.25,99.5));
#21173=CARTESIAN_POINT('',(210.,14.,75.8));
#21174=CARTESIAN_POINT('',(210.,14.,100.));
#21175=CARTESIAN_POINT('',(210.,14.3,75.5));
#21176=CARTESIAN_POINT('',(210.,24.4,65.4));
#21177=CARTESIAN_POINT('',(210.,36.5,75.5));
#21178=CARTESIAN_POINT('',(210.,14.,75.5));
#21179=CARTESIAN_POINT('',(210.,36.5,60.));
#21180=CARTESIAN_POINT('',(210.,36.5,75.5));
#21181=CARTESIAN_POINT('',(210.,32.,60.));
#21182=CARTESIAN_POINT('',(210.,36.5,60.));
#21183=CARTESIAN_POINT('',(210.,32.,40.));
#21184=CARTESIAN_POINT('',(210.,32.,60.));
#21185=CARTESIAN_POINT('',(210.,36.5,40.));
#21186=CARTESIAN_POINT('',(210.,32.,40.));
#21187=CARTESIAN_POINT('',(210.,36.5,24.5));
#21188=CARTESIAN_POINT('',(210.,36.5,40.));
#21189=CARTESIAN_POINT('',(210.,14.3,24.5));
#21190=CARTESIAN_POINT('',(210.,36.5,24.5));
#21191=CARTESIAN_POINT('',(210.,14.,24.2));
#21192=CARTESIAN_POINT('',(210.,24.4000000000001,34.5999999999999));
#21193=CARTESIAN_POINT('',(210.,14.,0.499999999999998));
#21194=CARTESIAN_POINT('',(210.,14.,24.5));
#21195=CARTESIAN_POINT('',(210.,44.5,0.499999999999998));
#21196=CARTESIAN_POINT('',(210.,21.75,0.499999999999998));
#21197=CARTESIAN_POINT('',(210.,44.5,25.));
#21198=CARTESIAN_POINT('',(210.,37.,22.35));
#21199=CARTESIAN_POINT('Origin',(210.,37.,20.));
#21200=CARTESIAN_POINT('',(210.,30.,6.35));
#21201=CARTESIAN_POINT('Origin',(210.,30.,4.));
#21202=CARTESIAN_POINT('',(210.,37.,82.35));
#21203=CARTESIAN_POINT('Origin',(210.,37.,80.));
#21204=CARTESIAN_POINT('Origin',(210.,30.,96.));
#21205=CARTESIAN_POINT('',(202.,30.,98.05));
#21206=CARTESIAN_POINT('',(210.,30.,98.05));
#21207=CARTESIAN_POINT('',(202.,27.95,96.));
#21208=CARTESIAN_POINT('Origin',(202.,30.,96.));
#21209=CARTESIAN_POINT('Origin',(202.,30.,96.));
#21210=CARTESIAN_POINT('Origin',(209.85,37.,20.));
#21211=CARTESIAN_POINT('',(209.7,37.,22.05));
#21212=CARTESIAN_POINT('Origin',(209.7,37.,20.));
#21213=CARTESIAN_POINT('',(209.85,37.,22.2));
#21214=CARTESIAN_POINT('Origin',(210.,37.,20.));
#21215=CARTESIAN_POINT('',(202.,37.,22.05));
#21216=CARTESIAN_POINT('',(210.,37.,22.05));
#21217=CARTESIAN_POINT('',(202.,34.95,20.));
#21218=CARTESIAN_POINT('Origin',(202.,37.,20.));
#21219=CARTESIAN_POINT('Origin',(202.,37.,20.));
#21220=CARTESIAN_POINT('Origin',(209.85,37.,80.));
#21221=CARTESIAN_POINT('',(209.7,37.,82.05));
#21222=CARTESIAN_POINT('Origin',(209.7,37.,80.));
#21223=CARTESIAN_POINT('',(209.85,37.,82.2));
#21224=CARTESIAN_POINT('Origin',(210.,37.,80.));
#21225=CARTESIAN_POINT('',(202.,37.,82.05));
#21226=CARTESIAN_POINT('',(210.,37.,82.05));
#21227=CARTESIAN_POINT('',(202.,34.95,80.));
#21228=CARTESIAN_POINT('Origin',(202.,37.,80.));
#21229=CARTESIAN_POINT('Origin',(202.,37.,80.));
#21230=CARTESIAN_POINT('Origin',(209.85,30.,4.));
#21231=CARTESIAN_POINT('',(209.7,30.,6.05));
#21232=CARTESIAN_POINT('Origin',(209.7,30.,4.));
#21233=CARTESIAN_POINT('',(209.85,30.,6.2));
#21234=CARTESIAN_POINT('Origin',(210.,30.,4.));
#21235=CARTESIAN_POINT('',(202.,30.,6.05));
#21236=CARTESIAN_POINT('',(210.,30.,6.05));
#21237=CARTESIAN_POINT('',(202.,27.95,4.));
#21238=CARTESIAN_POINT('Origin',(202.,30.,4.));
#21239=CARTESIAN_POINT('Origin',(202.,30.,4.));
#21240=CARTESIAN_POINT('Origin',(201.384117865497,30.,96.));
#21241=CARTESIAN_POINT('',(200.768235730993,30.,96.));
#21242=CARTESIAN_POINT('',(201.384117865497,28.975,96.));
#21243=CARTESIAN_POINT('Origin',(201.384117865497,30.,4.));
#21244=CARTESIAN_POINT('',(200.768235730993,30.,4.));
#21245=CARTESIAN_POINT('',(201.384117865497,28.975,4.));
#21246=CARTESIAN_POINT('Origin',(201.384117865497,37.,80.));
#21247=CARTESIAN_POINT('',(200.768235730993,37.,80.));
#21248=CARTESIAN_POINT('',(201.384117865497,35.975,80.));
#21249=CARTESIAN_POINT('Origin',(201.384117865497,37.,20.));
#21250=CARTESIAN_POINT('',(200.768235730993,37.,20.));
#21251=CARTESIAN_POINT('',(201.384117865497,35.975,20.));
#21252=CARTESIAN_POINT('Origin',(0.15,30.,96.));
#21253=CARTESIAN_POINT('',(0.3,30.,98.05));
#21254=CARTESIAN_POINT('Origin',(0.3,30.,96.));
#21255=CARTESIAN_POINT('',(0.,30.,98.35));
#21256=CARTESIAN_POINT('',(0.15,30.,98.2));
#21257=CARTESIAN_POINT('Origin',(0.,30.,96.));
#21258=CARTESIAN_POINT('Origin',(0.,29.5,50.));
#21259=CARTESIAN_POINT('',(0.,14.,0.499999999999998));
#21260=CARTESIAN_POINT('',(0.,44.5,0.499999999999998));
#21261=CARTESIAN_POINT('',(0.,21.75,0.499999999999998));
#21262=CARTESIAN_POINT('',(0.,14.,24.2));
#21263=CARTESIAN_POINT('',(0.,14.,24.5));
#21264=CARTESIAN_POINT('',(0.,14.3,24.5));
#21265=CARTESIAN_POINT('',(0.,24.4000000000001,34.5999999999999));
#21266=CARTESIAN_POINT('',(0.,36.5,24.5));
#21267=CARTESIAN_POINT('',(0.,36.5,24.5));
#21268=CARTESIAN_POINT('',(0.,36.5,40.));
#21269=CARTESIAN_POINT('',(0.,36.5,40.));
#21270=CARTESIAN_POINT('',(0.,32.,40.));
#21271=CARTESIAN_POINT('',(0.,32.,40.));
#21272=CARTESIAN_POINT('',(0.,32.,60.));
#21273=CARTESIAN_POINT('',(0.,32.,60.));
#21274=CARTESIAN_POINT('',(0.,36.5,60.));
#21275=CARTESIAN_POINT('',(0.,36.5,60.));
#21276=CARTESIAN_POINT('',(0.,36.5,75.5));
#21277=CARTESIAN_POINT('',(0.,36.5,75.5));
#21278=CARTESIAN_POINT('',(0.,14.3,75.5));
#21279=CARTESIAN_POINT('',(0.,14.,75.5));
#21280=CARTESIAN_POINT('',(0.,14.,75.8));
#21281=CARTESIAN_POINT('',(0.,24.4,65.4));
#21282=CARTESIAN_POINT('',(0.,14.,99.5));
#21283=CARTESIAN_POINT('',(0.,14.,100.));
#21284=CARTESIAN_POINT('',(0.,44.5,99.5));
#21285=CARTESIAN_POINT('',(0.,37.25,99.5));
#21286=CARTESIAN_POINT('',(0.,44.5,25.));
#21287=CARTESIAN_POINT('',(0.,37.,22.35));
#21288=CARTESIAN_POINT('Origin',(0.,37.,20.));
#21289=CARTESIAN_POINT('',(0.,30.,6.35));
#21290=CARTESIAN_POINT('Origin',(0.,30.,4.));
#21291=CARTESIAN_POINT('',(0.,37.,82.35));
#21292=CARTESIAN_POINT('Origin',(0.,37.,80.));
#21293=CARTESIAN_POINT('Origin',(0.,30.,96.));
#21294=CARTESIAN_POINT('',(8.,30.,98.05));
#21295=CARTESIAN_POINT('',(0.,30.,98.05));
#21296=CARTESIAN_POINT('',(7.99999999999999,27.95,96.));
#21297=CARTESIAN_POINT('Origin',(8.,30.,96.));
#21298=CARTESIAN_POINT('Origin',(8.,30.,96.));
#21299=CARTESIAN_POINT('Origin',(0.15,37.,20.));
#21300=CARTESIAN_POINT('',(0.3,37.,22.05));
#21301=CARTESIAN_POINT('Origin',(0.3,37.,20.));
#21302=CARTESIAN_POINT('',(0.15,37.,22.2));
#21303=CARTESIAN_POINT('Origin',(0.,37.,20.));
#21304=CARTESIAN_POINT('',(8.,37.,22.05));
#21305=CARTESIAN_POINT('',(0.,37.,22.05));
#21306=CARTESIAN_POINT('',(8.,34.95,20.));
#21307=CARTESIAN_POINT('Origin',(8.,37.,20.));
#21308=CARTESIAN_POINT('Origin',(8.,37.,20.));
#21309=CARTESIAN_POINT('Origin',(0.15,37.,80.));
#21310=CARTESIAN_POINT('',(0.3,37.,82.05));
#21311=CARTESIAN_POINT('Origin',(0.3,37.,80.));
#21312=CARTESIAN_POINT('',(0.15,37.,82.2));
#21313=CARTESIAN_POINT('Origin',(0.,37.,80.));
#21314=CARTESIAN_POINT('',(8.,37.,82.05));
#21315=CARTESIAN_POINT('',(0.,37.,82.05));
#21316=CARTESIAN_POINT('',(8.,34.95,80.));
#21317=CARTESIAN_POINT('Origin',(8.,37.,80.));
#21318=CARTESIAN_POINT('Origin',(8.,37.,80.));
#21319=CARTESIAN_POINT('Origin',(0.15,30.,4.));
#21320=CARTESIAN_POINT('',(0.3,30.,6.05));
#21321=CARTESIAN_POINT('Origin',(0.3,30.,4.));
#21322=CARTESIAN_POINT('',(0.15,30.,6.2));
#21323=CARTESIAN_POINT('Origin',(0.,30.,4.));
#21324=CARTESIAN_POINT('',(8.,30.,6.05));
#21325=CARTESIAN_POINT('',(0.,30.,6.05));
#21326=CARTESIAN_POINT('',(8.,27.95,4.));
#21327=CARTESIAN_POINT('Origin',(8.,30.,4.));
#21328=CARTESIAN_POINT('Origin',(8.,30.,4.));
#21329=CARTESIAN_POINT('Origin',(8.,30.,96.));
#21330=CARTESIAN_POINT('',(9.2317642690065,30.,96.));
#21331=CARTESIAN_POINT('',(8.,27.95,96.));
#21332=CARTESIAN_POINT('Origin',(8.,30.,4.));
#21333=CARTESIAN_POINT('',(9.2317642690065,30.,4.));
#21334=CARTESIAN_POINT('',(8.,27.95,4.));
#21335=CARTESIAN_POINT('Origin',(8.,37.,80.));
#21336=CARTESIAN_POINT('',(9.2317642690065,37.,80.));
#21337=CARTESIAN_POINT('',(8.,34.95,80.));
#21338=CARTESIAN_POINT('Origin',(8.,37.,20.));
#21339=CARTESIAN_POINT('',(9.2317642690065,37.,20.));
#21340=CARTESIAN_POINT('',(8.,34.95,20.));
#21341=CARTESIAN_POINT('Origin',(155.,44.8,75.));
#21342=CARTESIAN_POINT('',(151.95,44.6,75.));
#21343=CARTESIAN_POINT('Origin',(155.,44.6,75.));
#21344=CARTESIAN_POINT('',(151.55,45.,75.));
#21345=CARTESIAN_POINT('',(151.75,44.8,75.));
#21346=CARTESIAN_POINT('Origin',(155.,45.,75.));
#21347=CARTESIAN_POINT('Origin',(0.,45.,0.));
#21348=CARTESIAN_POINT('',(209.5,45.,0.5));
#21349=CARTESIAN_POINT('',(209.5,45.,99.5));
#21350=CARTESIAN_POINT('',(209.5,45.,25.));
#21351=CARTESIAN_POINT('',(0.5,45.,0.5));
#21352=CARTESIAN_POINT('',(0.,45.,0.5));
#21353=CARTESIAN_POINT('',(0.5,45.,99.5));
#21354=CARTESIAN_POINT('',(0.5,45.,25.));
#21355=CARTESIAN_POINT('',(0.,45.,99.5));
#21356=CARTESIAN_POINT('',(101.55,45.,75.));
#21357=CARTESIAN_POINT('Origin',(105.,45.,75.));
#21358=CARTESIAN_POINT('',(51.55,45.,75.));
#21359=CARTESIAN_POINT('Origin',(55.,45.,75.));
#21360=CARTESIAN_POINT('',(151.55,45.,25.));
#21361=CARTESIAN_POINT('Origin',(155.,45.,25.));
#21362=CARTESIAN_POINT('',(174.2,45.,81.5));
#21363=CARTESIAN_POINT('Origin',(180.,45.,81.5));
#21364=CARTESIAN_POINT('',(24.2,45.,18.5));
#21365=CARTESIAN_POINT('Origin',(30.,45.,18.5));
#21366=CARTESIAN_POINT('',(24.2,45.,81.5));
#21367=CARTESIAN_POINT('Origin',(30.,45.,81.5));
#21368=CARTESIAN_POINT('',(124.2,45.,18.5));
#21369=CARTESIAN_POINT('Origin',(130.,45.,18.5));
#21370=CARTESIAN_POINT('',(174.2,45.,18.5));
#21371=CARTESIAN_POINT('Origin',(180.,45.,18.5));
#21372=CARTESIAN_POINT('',(74.2,45.,81.5));
#21373=CARTESIAN_POINT('Origin',(80.,45.,81.5));
#21374=CARTESIAN_POINT('',(74.2,45.,18.5));
#21375=CARTESIAN_POINT('Origin',(80.,45.,18.5));
#21376=CARTESIAN_POINT('',(124.2,45.,81.5));
#21377=CARTESIAN_POINT('Origin',(130.,45.,81.5));
#21378=CARTESIAN_POINT('',(51.55,45.,25.));
#21379=CARTESIAN_POINT('Origin',(55.,45.,25.));
#21380=CARTESIAN_POINT('',(101.55,45.,25.));
#21381=CARTESIAN_POINT('Origin',(105.,45.,25.));
#21382=CARTESIAN_POINT('Origin',(155.,45.,75.));
#21383=CARTESIAN_POINT('',(151.95,38.5,75.));
#21384=CARTESIAN_POINT('',(151.95,45.,75.));
#21385=CARTESIAN_POINT('Origin',(155.,38.5,75.));
#21386=CARTESIAN_POINT('Origin',(105.,44.8,75.));
#21387=CARTESIAN_POINT('',(101.95,44.6,75.));
#21388=CARTESIAN_POINT('Origin',(105.,44.6,75.));
#21389=CARTESIAN_POINT('',(101.75,44.8,75.));
#21390=CARTESIAN_POINT('Origin',(105.,45.,75.));
#21391=CARTESIAN_POINT('',(101.95,38.5,75.));
#21392=CARTESIAN_POINT('',(101.95,45.,75.));
#21393=CARTESIAN_POINT('Origin',(105.,38.5,75.));
#21394=CARTESIAN_POINT('Origin',(105.,44.8,25.));
#21395=CARTESIAN_POINT('',(101.95,44.6,25.));
#21396=CARTESIAN_POINT('Origin',(105.,44.6,25.));
#21397=CARTESIAN_POINT('',(101.75,44.8,25.));
#21398=CARTESIAN_POINT('Origin',(105.,45.,25.));
#21399=CARTESIAN_POINT('',(101.95,38.5,25.));
#21400=CARTESIAN_POINT('',(101.95,45.,25.));
#21401=CARTESIAN_POINT('Origin',(105.,38.5,25.));
#21402=CARTESIAN_POINT('Origin',(55.,44.8,75.));
#21403=CARTESIAN_POINT('',(51.95,44.6,75.));
#21404=CARTESIAN_POINT('Origin',(55.,44.6,75.));
#21405=CARTESIAN_POINT('',(51.75,44.8,75.));
#21406=CARTESIAN_POINT('Origin',(55.,45.,75.));
#21407=CARTESIAN_POINT('',(51.95,38.5,75.));
#21408=CARTESIAN_POINT('',(51.95,45.,75.));
#21409=CARTESIAN_POINT('Origin',(55.,38.5,75.));
#21410=CARTESIAN_POINT('Origin',(55.,44.8,25.));
#21411=CARTESIAN_POINT('',(51.95,44.6,25.));
#21412=CARTESIAN_POINT('Origin',(55.,44.6,25.));
#21413=CARTESIAN_POINT('',(51.75,44.8,25.));
#21414=CARTESIAN_POINT('Origin',(55.,45.,25.));
#21415=CARTESIAN_POINT('',(51.95,38.5,25.));
#21416=CARTESIAN_POINT('',(51.95,45.,25.));
#21417=CARTESIAN_POINT('Origin',(55.,38.5,25.));
#21418=CARTESIAN_POINT('Origin',(155.,44.8,25.));
#21419=CARTESIAN_POINT('',(151.95,44.6,25.));
#21420=CARTESIAN_POINT('Origin',(155.,44.6,25.));
#21421=CARTESIAN_POINT('',(151.75,44.8,25.));
#21422=CARTESIAN_POINT('Origin',(155.,45.,25.));
#21423=CARTESIAN_POINT('',(151.95,38.5,25.));
#21424=CARTESIAN_POINT('',(151.95,45.,25.));
#21425=CARTESIAN_POINT('Origin',(155.,38.5,25.));
#21426=CARTESIAN_POINT('Origin',(155.,38.5,75.));
#21427=CARTESIAN_POINT('',(155.,36.6673751119659,75.));
#21428=CARTESIAN_POINT('',(151.95,38.5,75.));
#21429=CARTESIAN_POINT('Origin',(155.,38.5,25.));
#21430=CARTESIAN_POINT('',(155.,36.6673751119659,25.));
#21431=CARTESIAN_POINT('',(151.95,38.5,25.));
#21432=CARTESIAN_POINT('Origin',(105.,38.5,75.));
#21433=CARTESIAN_POINT('',(105.,36.6673751119659,75.));
#21434=CARTESIAN_POINT('',(101.95,38.5,75.));
#21435=CARTESIAN_POINT('Origin',(105.,38.5,25.));
#21436=CARTESIAN_POINT('',(105.,36.6673751119659,25.));
#21437=CARTESIAN_POINT('',(101.95,38.5,25.));
#21438=CARTESIAN_POINT('Origin',(55.,38.5,75.));
#21439=CARTESIAN_POINT('',(55.,36.6673751119659,75.));
#21440=CARTESIAN_POINT('',(51.95,38.5,75.));
#21441=CARTESIAN_POINT('Origin',(55.,38.5,25.));
#21442=CARTESIAN_POINT('',(55.,36.6673751119659,25.));
#21443=CARTESIAN_POINT('',(51.95,38.5,25.));
#21444=CARTESIAN_POINT('Origin',(180.,44.85,81.5));
#21445=CARTESIAN_POINT('',(174.5,44.7,81.5));
#21446=CARTESIAN_POINT('Origin',(180.,44.7,81.5));
#21447=CARTESIAN_POINT('',(174.35,44.85,81.5));
#21448=CARTESIAN_POINT('Origin',(180.,45.,81.5));
#21449=CARTESIAN_POINT('',(174.5,38.,81.5));
#21450=CARTESIAN_POINT('',(174.5,45.,81.5));
#21451=CARTESIAN_POINT('Origin',(180.,38.,81.5));
#21452=CARTESIAN_POINT('Origin',(130.,44.85,81.5));
#21453=CARTESIAN_POINT('',(124.5,44.7,81.5));
#21454=CARTESIAN_POINT('Origin',(130.,44.7,81.5));
#21455=CARTESIAN_POINT('',(124.35,44.85,81.5));
#21456=CARTESIAN_POINT('Origin',(130.,45.,81.5));
#21457=CARTESIAN_POINT('',(124.5,38.,81.5));
#21458=CARTESIAN_POINT('',(124.5,45.,81.5));
#21459=CARTESIAN_POINT('Origin',(130.,38.,81.5));
#21460=CARTESIAN_POINT('Origin',(30.,44.85,18.5));
#21461=CARTESIAN_POINT('',(24.5,44.7,18.5));
#21462=CARTESIAN_POINT('Origin',(30.,44.7,18.5));
#21463=CARTESIAN_POINT('',(24.35,44.85,18.5));
#21464=CARTESIAN_POINT('Origin',(30.,45.,18.5));
#21465=CARTESIAN_POINT('',(24.5,38.,18.5));
#21466=CARTESIAN_POINT('',(24.5,45.,18.5));
#21467=CARTESIAN_POINT('Origin',(30.,38.,18.5));
#21468=CARTESIAN_POINT('Origin',(80.,44.85,18.5));
#21469=CARTESIAN_POINT('',(74.5,44.7,18.5));
#21470=CARTESIAN_POINT('Origin',(80.,44.7,18.5));
#21471=CARTESIAN_POINT('',(74.35,44.85,18.5));
#21472=CARTESIAN_POINT('Origin',(80.,45.,18.5));
#21473=CARTESIAN_POINT('',(74.5,38.,18.5));
#21474=CARTESIAN_POINT('',(74.5,45.,18.5));
#21475=CARTESIAN_POINT('Origin',(80.,38.,18.5));
#21476=CARTESIAN_POINT('Origin',(30.,44.85,81.5));
#21477=CARTESIAN_POINT('',(24.5,44.7,81.5));
#21478=CARTESIAN_POINT('Origin',(30.,44.7,81.5));
#21479=CARTESIAN_POINT('',(24.35,44.85,81.5));
#21480=CARTESIAN_POINT('Origin',(30.,45.,81.5));
#21481=CARTESIAN_POINT('',(24.5,38.,81.5));
#21482=CARTESIAN_POINT('',(24.5,45.,81.5));
#21483=CARTESIAN_POINT('Origin',(30.,38.,81.5));
#21484=CARTESIAN_POINT('Origin',(80.,44.85,81.5));
#21485=CARTESIAN_POINT('',(74.5,44.7,81.5));
#21486=CARTESIAN_POINT('Origin',(80.,44.7,81.5));
#21487=CARTESIAN_POINT('',(74.35,44.85,81.5));
#21488=CARTESIAN_POINT('Origin',(80.,45.,81.5));
#21489=CARTESIAN_POINT('',(74.5,38.,81.5));
#21490=CARTESIAN_POINT('',(74.5,45.,81.5));
#21491=CARTESIAN_POINT('Origin',(80.,38.,81.5));
#21492=CARTESIAN_POINT('Origin',(130.,44.85,18.5));
#21493=CARTESIAN_POINT('',(124.5,44.7,18.5));
#21494=CARTESIAN_POINT('Origin',(130.,44.7,18.5));
#21495=CARTESIAN_POINT('',(124.35,44.85,18.5));
#21496=CARTESIAN_POINT('Origin',(130.,45.,18.5));
#21497=CARTESIAN_POINT('',(124.5,38.,18.5));
#21498=CARTESIAN_POINT('',(124.5,45.,18.5));
#21499=CARTESIAN_POINT('Origin',(130.,38.,18.5));
#21500=CARTESIAN_POINT('Origin',(180.,44.85,18.5));
#21501=CARTESIAN_POINT('',(174.5,44.7,18.5));
#21502=CARTESIAN_POINT('Origin',(180.,44.7,18.5));
#21503=CARTESIAN_POINT('',(174.35,44.85,18.5));
#21504=CARTESIAN_POINT('Origin',(180.,45.,18.5));
#21505=CARTESIAN_POINT('',(174.5,38.,18.5));
#21506=CARTESIAN_POINT('',(174.5,45.,18.5));
#21507=CARTESIAN_POINT('Origin',(180.,38.,18.5));
#21508=CARTESIAN_POINT('Origin',(180.,38.,18.5));
#21509=CARTESIAN_POINT('',(176.5,38.,18.5));
#21510=CARTESIAN_POINT('Origin',(180.,38.,18.5));
#21511=CARTESIAN_POINT('Origin',(130.,38.,18.5));
#21512=CARTESIAN_POINT('',(126.5,38.,18.5));
#21513=CARTESIAN_POINT('Origin',(130.,38.,18.5));
#21514=CARTESIAN_POINT('Origin',(80.,38.,81.5));
#21515=CARTESIAN_POINT('',(76.5,38.,81.5));
#21516=CARTESIAN_POINT('Origin',(80.,38.,81.5));
#21517=CARTESIAN_POINT('Origin',(30.,38.,81.5));
#21518=CARTESIAN_POINT('',(26.5,38.,81.5));
#21519=CARTESIAN_POINT('Origin',(30.,38.,81.5));
#21520=CARTESIAN_POINT('Origin',(80.,38.,18.5));
#21521=CARTESIAN_POINT('',(76.5,38.,18.5));
#21522=CARTESIAN_POINT('Origin',(80.,38.,18.5));
#21523=CARTESIAN_POINT('Origin',(30.,38.,18.5));
#21524=CARTESIAN_POINT('',(26.5,38.,18.5));
#21525=CARTESIAN_POINT('Origin',(30.,38.,18.5));
#21526=CARTESIAN_POINT('Origin',(130.,38.,81.5));
#21527=CARTESIAN_POINT('',(126.5,38.,81.5));
#21528=CARTESIAN_POINT('Origin',(130.,38.,81.5));
#21529=CARTESIAN_POINT('Origin',(180.,38.,81.5));
#21530=CARTESIAN_POINT('',(176.5,38.,81.5));
#21531=CARTESIAN_POINT('Origin',(180.,38.,81.5));
#21532=CARTESIAN_POINT('Origin',(180.,45.,18.5));
#21533=CARTESIAN_POINT('',(176.5,14.,18.5));
#21534=CARTESIAN_POINT('',(176.5,45.,18.5));
#21535=CARTESIAN_POINT('Origin',(180.,14.,18.5));
#21536=CARTESIAN_POINT('Origin',(130.,45.,18.5));
#21537=CARTESIAN_POINT('',(126.5,14.,18.5));
#21538=CARTESIAN_POINT('',(126.5,45.,18.5));
#21539=CARTESIAN_POINT('Origin',(130.,14.,18.5));
#21540=CARTESIAN_POINT('Origin',(80.,45.,81.5));
#21541=CARTESIAN_POINT('',(76.5,14.,81.5));
#21542=CARTESIAN_POINT('',(76.5,45.,81.5));
#21543=CARTESIAN_POINT('Origin',(80.,14.,81.5));
#21544=CARTESIAN_POINT('Origin',(30.,45.,81.5));
#21545=CARTESIAN_POINT('',(26.5,14.,81.5));
#21546=CARTESIAN_POINT('',(26.5,45.,81.5));
#21547=CARTESIAN_POINT('Origin',(30.,14.,81.5));
#21548=CARTESIAN_POINT('Origin',(80.,45.,18.5));
#21549=CARTESIAN_POINT('',(76.5,14.,18.5));
#21550=CARTESIAN_POINT('',(76.5,45.,18.5));
#21551=CARTESIAN_POINT('Origin',(80.,14.,18.5));
#21552=CARTESIAN_POINT('Origin',(30.,45.,18.5));
#21553=CARTESIAN_POINT('',(26.5,14.,18.5));
#21554=CARTESIAN_POINT('',(26.5,45.,18.5));
#21555=CARTESIAN_POINT('Origin',(30.,14.,18.5));
#21556=CARTESIAN_POINT('Origin',(130.,45.,81.5));
#21557=CARTESIAN_POINT('',(126.5,14.,81.5));
#21558=CARTESIAN_POINT('',(126.5,45.,81.5));
#21559=CARTESIAN_POINT('Origin',(130.,14.,81.5));
#21560=CARTESIAN_POINT('Origin',(180.,45.,81.5));
#21561=CARTESIAN_POINT('',(176.5,14.,81.5));
#21562=CARTESIAN_POINT('',(176.5,45.,81.5));
#21563=CARTESIAN_POINT('Origin',(180.,14.,81.5));
#21564=CARTESIAN_POINT('Origin',(209.75,37.25,99.75));
#21565=CARTESIAN_POINT('',(170.958333333333,53.0416666666664,138.541666666667));
#21566=CARTESIAN_POINT('',(209.75,44.75,99.75));
#21567=CARTESIAN_POINT('',(223.458333333333,31.0416666666668,86.0416666666665));
#21568=CARTESIAN_POINT('',(173.541666666667,8.54166666666666,135.958333333333));
#21569=CARTESIAN_POINT('Origin',(209.75,44.75,25.));
#21570=CARTESIAN_POINT('',(209.75,44.75,0.250000000000017));
#21571=CARTESIAN_POINT('',(217.708333333333,36.7916666666668,8.20833333333323));
#21572=CARTESIAN_POINT('',(170.666666666666,83.8333333333334,39.3333333333336));
#21573=CARTESIAN_POINT('',(162.333333333332,92.1666666666667,52.3333333333333));
#21574=CARTESIAN_POINT('Origin',(0.,14.25,99.75));
#21575=CARTESIAN_POINT('',(4.04166666666663,18.0416666666666,103.541666666667));
#21576=CARTESIAN_POINT('',(0.,14.,99.5));
#21577=CARTESIAN_POINT('Origin',(0.,44.75,0.25));
#21578=CARTESIAN_POINT('',(170.958333333332,5.95833333333323,-38.5416666666669));
#21579=CARTESIAN_POINT('',(0.249999999999999,44.75,0.250000000000001));
#21580=CARTESIAN_POINT('',(4.04166666666667,40.9583333333334,-3.54166666666665));
#21581=CARTESIAN_POINT('',(4.33333333333334,48.8333333333333,4.33333333333334));
#21582=CARTESIAN_POINT('Origin',(209.75,21.75,0.249999999999999));
#21583=CARTESIAN_POINT('',(173.541666666666,50.4583333333335,-35.9583333333336));
#21584=CARTESIAN_POINT('Origin',(0.25,21.75,0.249999999999999));
#21585=CARTESIAN_POINT('',(1.45833333333333,15.4583333333333,-0.958333333333329));
#21586=CARTESIAN_POINT('',(-7.70833333333334,36.7916666666667,8.20833333333331));
#21587=CARTESIAN_POINT('Origin',(0.25,44.75,25.));
#21588=CARTESIAN_POINT('',(0.25,44.75,99.75));
#21589=CARTESIAN_POINT('',(-13.4583333333334,31.0416666666666,86.0416666666664));
#21590=CARTESIAN_POINT('',(12.6666666666667,57.1666666666666,87.3333333333334));
#21591=CARTESIAN_POINT('Origin',(0.,44.75,99.75));
#21592=CARTESIAN_POINT('',(1.45833333333333,43.5416666666667,100.958333333333));
#21593=CARTESIAN_POINT('Origin',(0.25,37.25,99.75));
#21594=CARTESIAN_POINT('Origin',(0.,14.15,24.35));
#21595=CARTESIAN_POINT('',(0.,14.3,24.5));
#21596=CARTESIAN_POINT('',(0.,14.,24.2));
#21597=CARTESIAN_POINT('Origin',(0.,14.,24.5));
#21598=CARTESIAN_POINT('',(0.,14.,0.5));
#21599=CARTESIAN_POINT('Origin',(0.,14.15,75.65));
#21600=CARTESIAN_POINT('',(0.,14.,75.8));
#21601=CARTESIAN_POINT('',(0.,14.3,75.5));
#21602=CARTESIAN_POINT('Origin',(0.,14.,75.5));
#21603=CARTESIAN_POINT('',(0.,36.5,75.5));
#21604=CARTESIAN_POINT('Origin',(0.,14.25,0.25));
#21605=CARTESIAN_POINT('Origin',(0.,14.,100.));
#21606=CARTESIAN_POINT('Origin',(0.,36.5,24.5));
#21607=CARTESIAN_POINT('',(0.,36.5,24.5));
#21608=CARTESIAN_POINT('Origin',(0.,36.5,40.));
#21609=CARTESIAN_POINT('',(0.,36.5,40.));
#21610=CARTESIAN_POINT('Origin',(0.,32.,40.));
#21611=CARTESIAN_POINT('',(0.,32.,40.));
#21612=CARTESIAN_POINT('Origin',(0.,32.,60.));
#21613=CARTESIAN_POINT('',(0.,32.,60.));
#21614=CARTESIAN_POINT('Origin',(0.,36.5,60.));
#21615=CARTESIAN_POINT('',(0.,36.5,60.));
#21616=CARTESIAN_POINT('Origin',(0.,36.5,75.5));
#81019=UNCERTAINTY_MEASURE_WITH_UNIT(LENGTH_MEASURE(0.01),#81041,
'DISTANCE_ACCURACY_VALUE',
'Maximum model space distance between geometric entities at asserted c
onnectivities');
#81028=UNCERTAINTY_MEASURE_WITH_UNIT(LENGTH_MEASURE(0.01),#81041,
'DISTANCE_ACCURACY_VALUE',
'Maximum model space distance between geometric entities at asserted c
onnectivities');
#81031=(
GEOMETRIC_REPRESENTATION_CONTEXT(3)
GLOBAL_UNCERTAINTY_ASSIGNED_CONTEXT((#81019))
GLOBAL_UNIT_ASSIGNED_CONTEXT((#81041,#81043,#81044))
REPRESENTATION_CONTEXT('','3D')
);
#81040=(
GEOMETRIC_REPRESENTATION_CONTEXT(3)
GLOBAL_UNCERTAINTY_ASSIGNED_CONTEXT((#81028))
GLOBAL_UNIT_ASSIGNED_CONTEXT((#81041,#81043,#81044))
REPRESENTATION_CONTEXT('','3D')
);
#81041=(
LENGTH_UNIT()
NAMED_UNIT(*)
SI_UNIT(.MILLI.,.METRE.)
);
#81043=(
NAMED_UNIT(*)
PLANE_ANGLE_UNIT()
SI_UNIT($,.RADIAN.)
);
#81044=(
NAMED_UNIT(*)
SI_UNIT($,.STERADIAN.)
SOLID_ANGLE_UNIT()
);
#81047=SHAPE_DEFINITION_REPRESENTATION(#81058,#81131);
#81058=PRODUCT_DEFINITION_SHAPE('',$,#81143);
#81131=SHAPE_REPRESENTATION('',(#15327),#81031);
#81140=PRODUCT_DEFINITION_CONTEXT('part definition',#81175,'design');
#81143=PRODUCT_DEFINITION('Table - Top Sliding Stage Platform',
'Table - Top Sliding Stage Platform',#81154,#81140);
#81154=PRODUCT_DEFINITION_FORMATION('',$,#81179);
#81175=APPLICATION_CONTEXT(
'Core Data for Automotive Mechanical Design Process');
#81176=PRODUCT_CONTEXT('part definition',#81175,'mechanical');
#81179=PRODUCT('Table - Top Sliding Stage Platform',
'Table - Top Sliding Stage Platform',$,(#81176));
#81190=PRESENTATION_STYLE_ASSIGNMENT((#81201));
#81201=SURFACE_STYLE_USAGE(.BOTH.,#81212);
#81212=SURFACE_SIDE_STYLE('',(#81223));
#81223=SURFACE_STYLE_FILL_AREA(#81234);
#81234=FILL_AREA_STYLE('Opaque(222,225,230)',(#81245));
#81245=FILL_AREA_STYLE_COLOUR('Opaque(222,225,230)',#81256);
#81256=COLOUR_RGB('Opaque(222,225,230)', 0.66274510, 0.83137255, 0.94901961);
ENDSEC;
END-ISO-10303-21;
